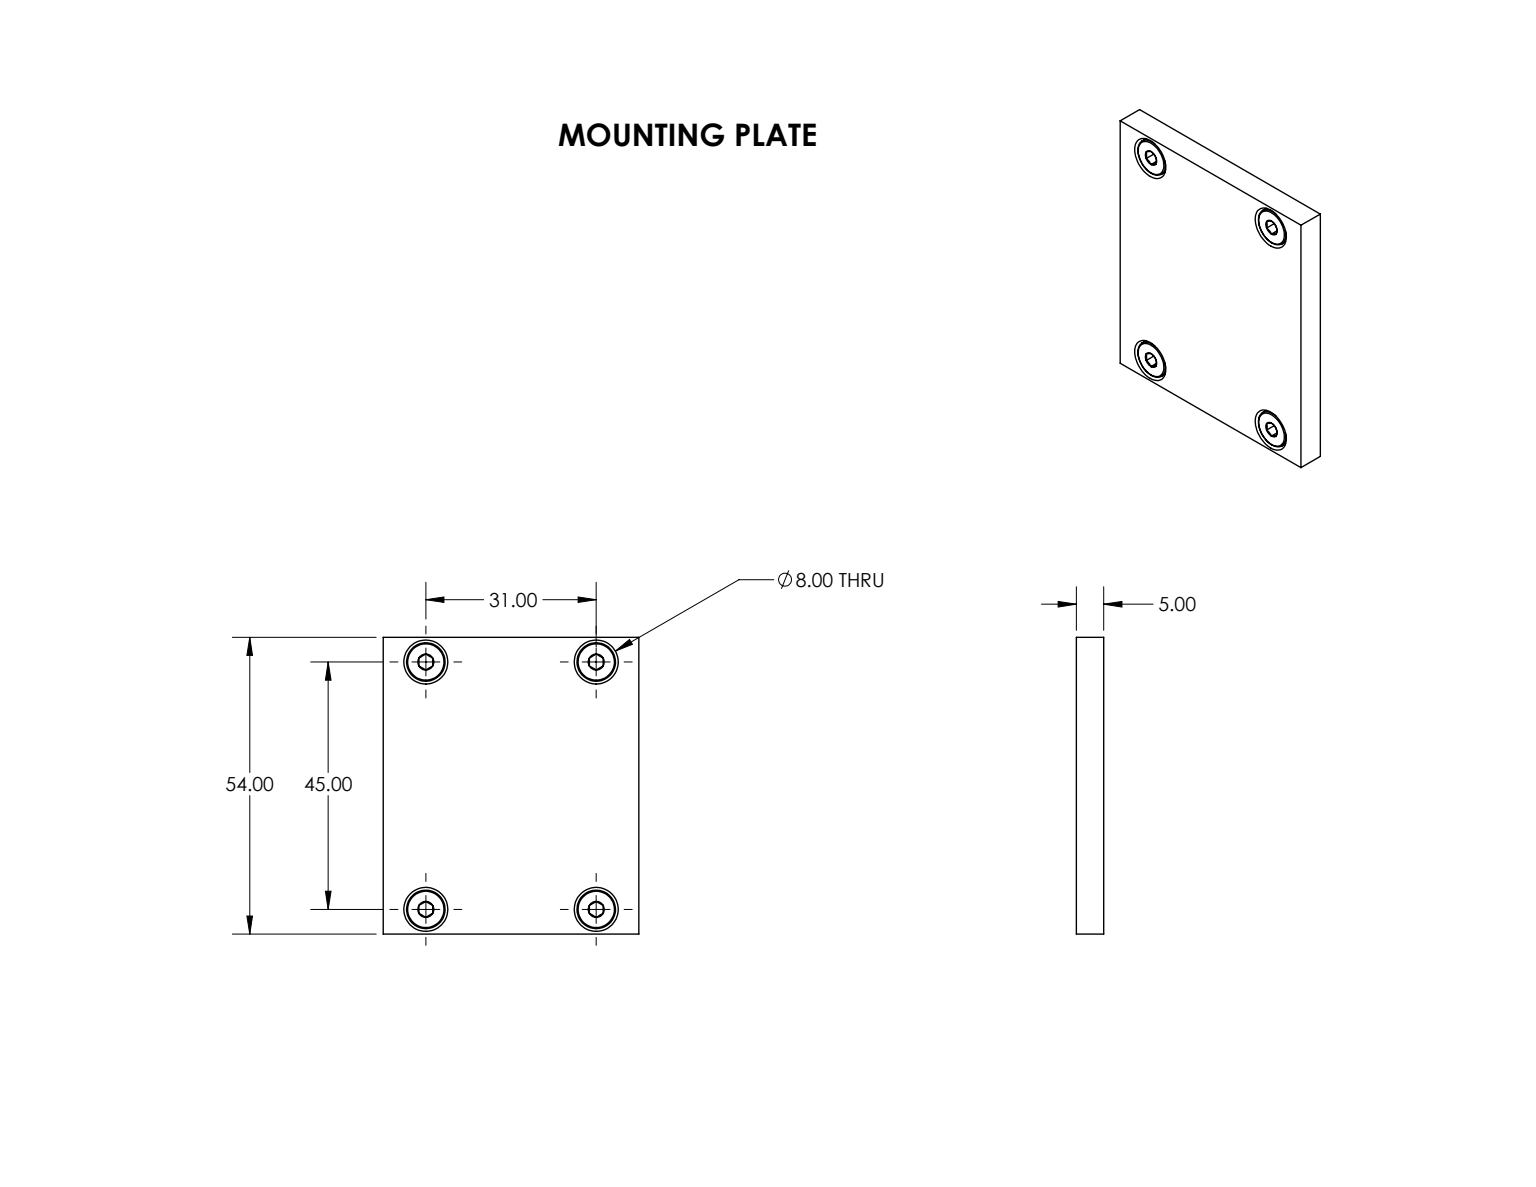
ISO-10303-21;
HEADER;
FILE_DESCRIPTION (('STEP AP214'),
    '1' );
FILE_NAME ('Mounting Plate.step',
    '2026-10-09T17:48:21',
    ( '' ),
    ( '' ),
    'SwSTEP 2.0',
    'SolidWorks 2024',
    '' );
FILE_SCHEMA (( 'AUTOMOTIVE_DESIGN' ));
ENDSEC;

DATA;
#5=CARTESIAN_POINT ( 'NONE',  ( -15.70313394609757296, -0.2715358723600092006, -23.82609623451302028 ) ) ;
#6=DIRECTION ( 'NONE',  ( 0.000000000000000000, 1.000000000000000000, 0.000000000000000000 ) ) ;
#12=DIRECTION ( 'NONE',  ( 0.000000000000000000, 0.000000000000000000, 1.000000000000000000 ) ) ;
#26=CARTESIAN_POINT ( 'NONE',  ( 14.25000000000000000, -0.2038245569916330158, 23.22168783648699986 ) ) ;
#31=CIRCLE ( 'NONE', #14646, 3.499999999999999556 ) ;
#37=ORIENTED_EDGE ( 'NONE', *, *, #9789, .F. ) ;
#41=CARTESIAN_POINT ( 'NONE',  ( 15.50000000000000000, -0.4000000000000000222, -22.50000000000000000 ) ) ;
#49=VECTOR ( 'NONE', #15077, 1000.000000000000000 ) ;
#51=VERTEX_POINT ( 'NONE', #8286 ) ;
#59=VERTEX_POINT ( 'NONE', #14253 ) ;
#64=CARTESIAN_POINT ( 'NONE',  ( -14.25000000000000000, -2.500000000000000000, -23.22168783648699986 ) ) ;
#66=DIRECTION ( 'NONE',  ( -0.8660254037844482555, 0.000000000000000000, 0.4999999999999831801 ) ) ;
#71=VERTEX_POINT ( 'NONE', #12157 ) ;
#76=CARTESIAN_POINT ( 'NONE',  ( -15.91242688423474050, -0.3152598339554945062, -23.70526090034005051 ) ) ;
#77=CARTESIAN_POINT ( 'NONE',  ( 15.50000000000000000, -2.500000000000000000, -21.05662432702600029 ) ) ;
#80=AXIS2_PLACEMENT_3D ( 'NONE', #7760, #5130, #12410 ) ;
#85=CARTESIAN_POINT ( 'NONE',  ( -14.66434062215826017, -0.3156604612126701626, -21.53909249377373669 ) ) ;
#93=AXIS2_PLACEMENT_3D ( 'NONE', #13950, #3324, #14805 ) ;
#96=ORIENTED_EDGE ( 'NONE', *, *, #11121, .T. ) ;
#98=DIRECTION ( 'NONE',  ( 0.000000000000000000, 1.000000000000000000, 0.000000000000000000 ) ) ;
#109=LINE ( 'NONE', #5963, #14166 ) ;
#122=FACE_OUTER_BOUND ( 'NONE', #15028, .T. ) ;
#123=DIRECTION ( 'NONE',  ( 0.000000000000000000, 1.000000000000000000, 0.000000000000000000 ) ) ;
#130=ORIENTED_EDGE ( 'NONE', *, *, #9024, .T. ) ;
#139=CARTESIAN_POINT ( 'NONE',  ( -16.75000000000000000, -2.500000000000000000, -23.22168783648699986 ) ) ;
#146=( NAMED_UNIT ( * ) SI_UNIT ( $, .STERADIAN. ) SOLID_ANGLE_UNIT ( ) );
#150=FACE_OUTER_BOUND ( 'NONE', #9608, .T. ) ;
#154=VECTOR ( 'NONE', #6765, 1000.000000000000000 ) ;
#164=DIRECTION ( 'NONE',  ( -0.9375000000000006661, 0.000000000000000000, -0.3479852726768744020 ) ) ;
#178=DIRECTION ( 'NONE',  ( 0.000000000000000000, 1.000000000000000000, 0.000000000000000000 ) ) ;
#181=VERTEX_POINT ( 'NONE', #14626 ) ;
#183=CARTESIAN_POINT ( 'NONE',  ( -15.50000000000000000, -5.000000000000000000, -22.50000000000000000 ) ) ;
#186=CIRCLE ( 'NONE', #13087, 4.000000000000000000 ) ;
#189=CARTESIAN_POINT ( 'NONE',  ( 15.50000000000000000, -0.4000000000000000222, 25.99999999999999645 ) ) ;
#203=DIRECTION ( 'NONE',  ( 0.000000000000000000, 1.000000000000000000, 0.000000000000000000 ) ) ;
#214=EDGE_CURVE ( 'NONE', #71, #6831, #12240, .T. ) ;
#215=VERTEX_POINT ( 'NONE', #12398 ) ;
#216=CIRCLE ( 'NONE', #8155, 3.499999999999999556 ) ;
#219=CARTESIAN_POINT ( 'NONE',  ( -23.24999999999999645, -5.000000000000000000, 2.987579319737834353E-15 ) ) ;
#240=LINE ( 'NONE', #14588, #11040 ) ;
#252=DIRECTION ( 'NONE',  ( 0.000000000000000000, 1.000000000000000000, 0.000000000000000000 ) ) ;
#253=CYLINDRICAL_SURFACE ( 'NONE', #1029, 4.000000000000000000 ) ;
#254=B_SPLINE_CURVE_WITH_KNOTS ( 'NONE', 3,
 ( #13370, #13070, #7240, #85, #9698, #9626 ),
 .UNSPECIFIED., .F., .F.,
 ( 4, 2, 4 ),
 ( 0.0002380763768129734448, 0.7291065797294584705, 1.457975083082104106 ),
 .UNSPECIFIED. ) ;
#256=DIRECTION ( 'NONE',  ( 0.000000000000000000, 0.000000000000000000, 1.000000000000000000 ) ) ;
#258=ORIENTED_EDGE ( 'NONE', *, *, #13416, .T. ) ;
#266=DIRECTION ( 'NONE',  ( 0.000000000000000000, 1.000000000000000000, 0.000000000000000000 ) ) ;
#272=CARTESIAN_POINT ( 'NONE',  ( 15.50000000000000000, 0.000000000000000000, 22.50000000000000000 ) ) ;
#273=PLANE ( 'NONE',  #3768 ) ;
#278=ORIENTED_EDGE ( 'NONE', *, *, #3265, .F. ) ;
#281=ORIENTED_EDGE ( 'NONE', *, *, #748, .F. ) ;
#285=AXIS2_PLACEMENT_3D ( 'NONE', #3423, #3496, #1409 ) ;
#298=MANIFOLD_SOLID_BREP ( 'Cut-Extrude1[3]', #2333 ) ;
#314=CARTESIAN_POINT ( 'NONE',  ( -15.50000000000000000, -0.4000000000000000222, -22.50000000000000000 ) ) ;
#330=MANIFOLD_SOLID_BREP ( 'Cut-Extrude1[2]', #3578 ) ;
#335=AXIS2_PLACEMENT_3D ( 'NONE', #8151, #10623, #9451 ) ;
#339=EDGE_CURVE ( 'NONE', #3097, #10442, #10612, .T. ) ;
#341=ORIENTED_EDGE ( 'NONE', *, *, #3984, .F. ) ;
#345=EDGE_CURVE ( 'NONE', #11913, #11111, #14089, .T. ) ;
#356=PLANE ( 'NONE',  #3581 ) ;
#363=ORIENTED_EDGE ( 'NONE', *, *, #4204, .F. ) ;
#382=VERTEX_POINT ( 'NONE', #12076 ) ;
#395=( NAMED_UNIT ( * ) SI_UNIT ( $, .STERADIAN. ) SOLID_ANGLE_UNIT ( ) );
#408=VECTOR ( 'NONE', #14676, 1000.000000000000000 ) ;
#412=ORIENTED_EDGE ( 'NONE', *, *, #7830, .T. ) ;
#429=AXIS2_PLACEMENT_3D ( 'NONE', #8275, #13100, #14013 ) ;
#446=DIRECTION ( 'NONE',  ( 0.000000000000000000, 0.000000000000000000, 1.000000000000000000 ) ) ;
#473=DIRECTION ( 'NONE',  ( 0.000000000000000000, 1.000000000000000000, 0.000000000000000000 ) ) ;
#475=PRESENTATION_STYLE_ASSIGNMENT (( #11957 ) ) ;
#481=CARTESIAN_POINT ( 'NONE',  ( -14.25000000000000000, -0.2038245569916330158, 23.22168783648699986 ) ) ;
#490=EDGE_CURVE ( 'NONE', #215, #4608, #7344, .T. ) ;
#496=DIRECTION ( 'NONE',  ( 0.000000000000000000, 1.000000000000000000, 0.000000000000000000 ) ) ;
#500=CARTESIAN_POINT ( 'NONE',  ( 14.25000000000000000, -2.500000000000000000, 23.22168783648699986 ) ) ;
#512=PLANE ( 'NONE',  #4120 ) ;
#523=ORIENTED_EDGE ( 'NONE', *, *, #11573, .T. ) ;
#528=CARTESIAN_POINT ( 'NONE',  ( -15.50000000000000000, -1.037157890325000054, 26.50000000000000000 ) ) ;
#531=FACE_OUTER_BOUND ( 'NONE', #5335, .T. ) ;
#535=DIRECTION ( 'NONE',  ( 0.000000000000000000, 0.000000000000000000, 1.000000000000000000 ) ) ;
#541=VERTEX_POINT ( 'NONE', #8623 ) ;
#544=FACE_OUTER_BOUND ( 'NONE', #4192, .T. ) ;
#552=CARTESIAN_POINT ( 'NONE',  ( -14.25000000000000000, -2.500000000000000000, 23.22168783648699986 ) ) ;
#553=CARTESIAN_POINT ( 'NONE',  ( -15.50000000000000000, -1.037157890325000054, -19.00000000000000000 ) ) ;
#562=CARTESIAN_POINT ( 'NONE',  ( 15.50000000000000000, -1.037157890325000054, -26.50000000000000000 ) ) ;
#579=CIRCLE ( 'NONE', #11243, 1.449999999999996403 ) ;
#580=EDGE_CURVE ( 'NONE', #13163, #4486, #254, .T. ) ;
#581=CIRCLE ( 'NONE', #80, 3.499999999999999556 ) ;
#589=DIRECTION ( 'NONE',  ( 0.000000000000000000, 0.5000000000000199840, 0.8660254037844271613 ) ) ;
#593=AXIS2_PLACEMENT_3D ( 'NONE', #5582, #6516, #11379 ) ;
#594=CARTESIAN_POINT ( 'NONE',  ( 15.50000000000000000, -5.000000000000000000, -19.00000000000000000 ) ) ;
#595=EDGE_CURVE ( 'NONE', #13129, #8137, #10804, .T. ) ;
#608=ORIENTED_EDGE ( 'NONE', *, *, #10263, .T. ) ;
#618=CARTESIAN_POINT ( 'NONE',  ( 14.25000000000000000, -0.2038245569916330158, -21.77831216351300014 ) ) ;
#621=ADVANCED_FACE ( 'NONE', ( #4203 ), #625, .F. ) ;
#625=PLANE ( 'NONE',  #12545 ) ;
#626=PRODUCT_DEFINITION_SHAPE ( 'NONE', 'NONE',  #15168 ) ;
#627=CARTESIAN_POINT ( 'NONE',  ( -15.50000000000000000, -0.2038245569916614930, -21.05662432702600029 ) ) ;
#634=VECTOR ( 'NONE', #10290, 1000.000000000000000 ) ;
#647=DIRECTION ( 'NONE',  ( -0.8660254037844485886, 0.000000000000000000, -0.4999999999999827360 ) ) ;
#649=CARTESIAN_POINT ( 'NONE',  ( 15.50000000000000000, -0.2000000000000000111, 25.80000000297970075 ) ) ;
#650=ORIENTED_EDGE ( 'NONE', *, *, #14893, .F. ) ;
#656=AXIS2_PLACEMENT_3D ( 'NONE', #9390, #1174, #6005 ) ;
#659=LINE ( 'NONE', #5414, #2818 ) ;
#660=CIRCLE ( 'NONE', #12071, 3.499999999999999556 ) ;
#662=DIRECTION ( 'NONE',  ( 0.000000000000000000, 0.000000000000000000, 1.000000000000000000 ) ) ;
#671=ORIENTED_EDGE ( 'NONE', *, *, #799, .F. ) ;
#674=CIRCLE ( 'NONE', #1917, 4.000000000000000000 ) ;
#679=CARTESIAN_POINT ( 'NONE',  ( 15.50000000000000000, -2.500000000000000000, -21.05662432702600029 ) ) ;
#680=CARTESIAN_POINT ( 'NONE',  ( 14.25000000000000000, -2.500000000000000000, -21.77831216351300014 ) ) ;
#687=EDGE_LOOP ( 'NONE', ( #7655, #1654 ) ) ;
#703=CARTESIAN_POINT ( 'NONE',  ( -15.91434062215688350, -0.3156604612129211285, -21.29584399676446793 ) ) ;
#728=ORIENTED_EDGE ( 'NONE', *, *, #5464, .T. ) ;
#733=DIRECTION ( 'NONE',  ( 0.000000000000000000, 0.000000000000000000, 1.000000000000000000 ) ) ;
#736=FACE_OUTER_BOUND ( 'NONE', #12730, .T. ) ;
#747=CARTESIAN_POINT ( 'NONE',  ( 15.50000000000000000, -1.037157890325000054, 22.50000000000000000 ) ) ;
#748=EDGE_CURVE ( 'NONE', #59, #4906, #2885, .T. ) ;
#761=DIRECTION ( 'NONE',  ( 0.000000000000000000, 1.000000000000000000, 0.000000000000000000 ) ) ;
#770=CARTESIAN_POINT ( 'NONE',  ( 16.75000000000000000, -0.2714405302574886547, 22.01253933645462624 ) ) ;
#777=VERTEX_POINT ( 'NONE', #6467 ) ;
#796=STYLED_ITEM ( 'NONE', ( #8444 ), #10531 ) ;
#799=EDGE_CURVE ( 'NONE', #1408, #5494, #8855, .T. ) ;
#805=EDGE_CURVE ( 'NONE', #71, #7389, #9667, .T. ) ;
#808=FACE_OUTER_BOUND ( 'NONE', #14949, .T. ) ;
#823=CARTESIAN_POINT ( 'NONE',  ( -16.94999999999999929, -0.2000000000000000111, -22.50000000000000000 ) ) ;
#825=CARTESIAN_POINT ( 'NONE',  ( 16.75000000000000000, -2.500000000000000000, -23.22168783648699986 ) ) ;
#833=VECTOR ( 'NONE', #8086, 1000.000000000000000 ) ;
#860=DIRECTION ( 'NONE',  ( 0.000000000000000000, 0.000000000000000000, -1.000000000000000000 ) ) ;
#868=DIRECTION ( 'NONE',  ( 0.000000000000000000, 0.000000000000000000, -1.000000000000000000 ) ) ;
#873=EDGE_LOOP ( 'NONE', ( #4886, #278 ) ) ;
#891=FACE_OUTER_BOUND ( 'NONE', #14981, .T. ) ;
#907=FACE_OUTER_BOUND ( 'NONE', #7178, .T. ) ;
#908=DIRECTION ( 'NONE',  ( 0.000000000000000000, 1.000000000000000000, 0.000000000000000000 ) ) ;
#915=ORIENTED_EDGE ( 'NONE', *, *, #5346, .F. ) ;
#931=ORIENTED_EDGE ( 'NONE', *, *, #748, .T. ) ;
#932=CARTESIAN_POINT ( 'NONE',  ( -14.25000000000000000, -0.2038245569916330158, -23.22168783648699986 ) ) ;
#933=ORIENTED_EDGE ( 'NONE', *, *, #4607, .F. ) ;
#938=LINE ( 'NONE', #14971, #4017 ) ;
#960=CARTESIAN_POINT ( 'NONE',  ( 15.50000000000000000, -0.4000000000005274892, -25.79999999999946780 ) ) ;
#961=CARTESIAN_POINT ( 'NONE',  ( -15.50000000000000000, -5.000000000000000000, -26.00000000000000000 ) ) ;
#965=ORIENTED_EDGE ( 'NONE', *, *, #6895, .T. ) ;
#966=DIRECTION ( 'NONE',  ( 0.000000000000000000, -1.000000000000000000, -0.000000000000000000 ) ) ;
#967=EDGE_CURVE ( 'NONE', #10723, #12753, #13779, .T. ) ;
#973=ORIENTED_EDGE ( 'NONE', *, *, #13857, .F. ) ;
#984=PLANE ( 'NONE',  #7031 ) ;
#986=ORIENTED_EDGE ( 'NONE', *, *, #6710, .F. ) ;
#996=FACE_OUTER_BOUND ( 'NONE', #7197, .T. ) ;
#997=EDGE_CURVE ( 'NONE', #8110, #14910, #1607, .T. ) ;
#1009=EDGE_LOOP ( 'NONE', ( #14869, #9513, #7261, #3118 ) ) ;
#1029=AXIS2_PLACEMENT_3D ( 'NONE', #10896, #5000, #9714 ) ;
#1038=CIRCLE ( 'NONE', #9708, 4.000000000000000000 ) ;
#1059=DIRECTION ( 'NONE',  ( 0.000000000000000000, 0.000000000000000000, 1.000000000000000000 ) ) ;
#1070=EDGE_CURVE ( 'NONE', #4318, #8552, #8080, .T. ) ;
#1072=DIRECTION ( 'NONE',  ( 0.000000000000000000, -0.000000000000000000, 1.000000000000000000 ) ) ;
#1073=DIRECTION ( 'NONE',  ( -0.4999999999999832356, 0.000000000000000000, -0.8660254037844483666 ) ) ;
#1075=B_SPLINE_CURVE_WITH_KNOTS ( 'NONE', 3,
 ( #9010, #12658, #3045, #2027, #15050, #12813 ),
 .UNSPECIFIED., .F., .F.,
 ( 4, 2, 4 ),
 ( 0.0002380763768129734448, 0.7291065797294589146, 1.457975083082104995 ),
 .UNSPECIFIED. ) ;
#1094=AXIS2_PLACEMENT_3D ( 'NONE', #12697, #4639, #6961 ) ;
#1095=EDGE_CURVE ( 'NONE', #11388, #11166, #13173, .T. ) ;
#1099=CARTESIAN_POINT ( 'NONE',  ( -14.25000000000000000, -0.2038245569916330158, 23.22168783648699986 ) ) ;
#1102=CARTESIAN_POINT ( 'NONE',  ( 16.75000000000000000, -2.500000000000000000, 21.77831216351300014 ) ) ;
#1109=ORIENTED_EDGE ( 'NONE', *, *, #4097, .F. ) ;
#1112=EDGE_CURVE ( 'NONE', #4275, #181, #10269, .T. ) ;
#1114=VERTEX_POINT ( 'NONE', #12546 ) ;
#1116=CARTESIAN_POINT ( 'NONE',  ( 15.50000000000000000, 0.000000000000000000, -22.50000000000000000 ) ) ;
#1118=AXIS2_PLACEMENT_3D ( 'NONE', #3027, #10142, #13735 ) ;
#1120=VECTOR ( 'NONE', #11401, 1000.000000000000000 ) ;
#1141=DIRECTION ( 'NONE',  ( 0.000000000000000000, 1.000000000000000000, 0.000000000000000000 ) ) ;
#1146=ORIENTED_EDGE ( 'NONE', *, *, #9815, .F. ) ;
#1150=EDGE_LOOP ( 'NONE', ( #965, #3065, #8473, #1387, #1741, #5883 ) ) ;
#1152=VECTOR ( 'NONE', #13066, 1000.000000000000000 ) ;
#1161=EDGE_CURVE ( 'NONE', #6610, #6972, #7948, .T. ) ;
#1166=CARTESIAN_POINT ( 'NONE',  ( -14.45313394609757118, -0.2715358723599894386, -23.33896727494798284 ) ) ;
#1168=ORIENTED_EDGE ( 'NONE', *, *, #4774, .F. ) ;
#1169=ORIENTED_EDGE ( 'NONE', *, *, #7747, .F. ) ;
#1173=EDGE_CURVE ( 'NONE', #1706, #5891, #11563, .T. ) ;
#1174=DIRECTION ( 'NONE',  ( -1.000000000000000000, 0.000000000000000000, 0.000000000000000000 ) ) ;
#1184=VERTEX_POINT ( 'NONE', #12393 ) ;
#1211=LINE ( 'NONE', #5970, #14749 ) ;
#1217=PLANE ( 'NONE',  #12937 ) ;
#1228=CARTESIAN_POINT ( 'NONE',  ( -30.00000000000000000, -5.000000000000000000, 27.00000000000000000 ) ) ;
#1229=DIRECTION ( 'NONE',  ( -0.000000000000000000, 1.000000000000000000, 0.000000000000000000 ) ) ;
#1246=LINE ( 'NONE', #4832, #3529 ) ;
#1254=ORIENTED_EDGE ( 'NONE', *, *, #1173, .F. ) ;
#1264=CARTESIAN_POINT ( 'NONE',  ( -16.33565937784310762, -0.3156604612129118026, 21.53909249377453250 ) ) ;
#1267=AXIS2_PLACEMENT_3D ( 'NONE', #823, #11377, #6737 ) ;
#1279=ORIENTED_EDGE ( 'NONE', *, *, #2419, .F. ) ;
#1280=AXIS2_PLACEMENT_3D ( 'NONE', #10048, #1980, #4088 ) ;
#1289=CARTESIAN_POINT ( 'NONE',  ( 14.25000000000000000, -2.500000000000000000, 23.22168783648699986 ) ) ;
#1309=FILL_AREA_STYLE ('',( #6070 ) ) ;
#1316=EDGE_LOOP ( 'NONE', ( #6456, #4036, #931, #1168 ) ) ;
#1318=ORIENTED_EDGE ( 'NONE', *, *, #12388, .T. ) ;
#1322=CARTESIAN_POINT ( 'NONE',  ( 15.50000000000000000, -5.000000000000000000, 22.50000000000000000 ) ) ;
#1324=AXIS2_PLACEMENT_3D ( 'NONE', #14681, #1434, #256 ) ;
#1332=CARTESIAN_POINT ( 'NONE',  ( -14.25000000000000000, -2.500000000000000000, 23.22168783648699986 ) ) ;
#1335=EDGE_CURVE ( 'NONE', #14415, #13870, #660, .T. ) ;
#1340=CLOSED_SHELL ( 'NONE', ( #1484, #14239, #7741, #10570, #14326, #4894, #5553, #4994, #9912, #11153, #4510, #6147, #11998, #6486 ) ) ;
#1359=EDGE_CURVE ( 'NONE', #3822, #12945, #13090, .T. ) ;
#1362=VECTOR ( 'NONE', #3810, 1000.000000000000000 ) ;
#1368=CARTESIAN_POINT ( 'NONE',  ( 14.25000000000000000, -2.500000000000000000, 21.77831216351300014 ) ) ;
#1387=ORIENTED_EDGE ( 'NONE', *, *, #1161, .T. ) ;
#1392=VECTOR ( 'NONE', #2531, 1000.000000000000000 ) ;
#1394=CARTESIAN_POINT ( 'NONE',  ( -15.50000000000000000, -5.000000000000000000, 19.00000000000000000 ) ) ;
#1408=VERTEX_POINT ( 'NONE', #5169 ) ;
#1409=DIRECTION ( 'NONE',  ( 1.000000000000000000, 0.000000000000000000, 0.000000000000000000 ) ) ;
#1418=FACE_OUTER_BOUND ( 'NONE', #5044, .T. ) ;
#1423=ORIENTED_EDGE ( 'NONE', *, *, #1112, .F. ) ;
#1424=ORIENTED_EDGE ( 'NONE', *, *, #4905, .F. ) ;
#1425=CARTESIAN_POINT ( 'NONE',  ( 15.50000000000000000, -0.2000000000000000111, 19.19999999702029925 ) ) ;
#1434=DIRECTION ( 'NONE',  ( 0.000000000000000000, -1.000000000000000000, -0.000000000000000000 ) ) ;
#1438=ORIENTED_EDGE ( 'NONE', *, *, #8297, .F. ) ;
#1439=DIRECTION ( 'NONE',  ( 0.000000000000000000, 1.000000000000000000, 0.000000000000000000 ) ) ;
#1443=EDGE_LOOP ( 'NONE', ( #933, #5709, #3137, #8529 ) ) ;
#1467=CIRCLE ( 'NONE', #10121, 3.499999999999999556 ) ;
#1476=ORIENTED_EDGE ( 'NONE', *, *, #3651, .F. ) ;
#1479=ADVANCED_FACE ( 'NONE', ( #2743 ), #8837, .T. ) ;
#1484=ADVANCED_FACE ( 'NONE', ( #8417 ), #13159, .F. ) ;
#1485=DIRECTION ( 'NONE',  ( 0.000000000000000000, 1.000000000000000000, 0.000000000000000000 ) ) ;
#1495=DIRECTION ( 'NONE',  ( 0.3479852726768751237, 0.000000000000000000, -0.9375000000000004441 ) ) ;
#1511=ORIENTED_EDGE ( 'NONE', *, *, #2723, .F. ) ;
#1512=VECTOR ( 'NONE', #13696, 1000.000000000000000 ) ;
#1519=CARTESIAN_POINT ( 'NONE',  ( -15.50000000000000000, -0.4000000000000000222, -19.00000000000000355 ) ) ;
#1522=PLANE ( 'NONE',  #10361 ) ;
#1528=VERTEX_POINT ( 'NONE', #189 ) ;
#1539=DIRECTION ( 'NONE',  ( 0.000000000000000000, 1.000000000000000000, 0.000000000000000000 ) ) ;
#1540=AXIS2_PLACEMENT_3D ( 'NONE', #14942, #4334, #13798 ) ;
#1551=VERTEX_POINT ( 'NONE', #649 ) ;
#1553=EDGE_CURVE ( 'NONE', #15023, #5866, #5990, .T. ) ;
#1559=CARTESIAN_POINT ( 'NONE',  ( 16.33757311576526305, -0.3152598339554795182, 21.54019739087904384 ) ) ;
#1607=LINE ( 'NONE', #5184, #9066 ) ;
#1610=EDGE_LOOP ( 'NONE', ( #8334, #14233 ) ) ;
#1620=PLANE ( 'NONE',  #12693 ) ;
#1628=VERTEX_POINT ( 'NONE', #500 ) ;
#1633=TOROIDAL_SURFACE ( 'NONE', #7823, 3.299999999999474909, 0.2000000000005234813 ) ;
#1635=AXIS2_PLACEMENT_3D ( 'NONE', #11045, #4929, #12135 ) ;
#1647=CARTESIAN_POINT ( 'NONE',  ( 16.75000000000000000, -0.2038245569916320166, -21.77831216351300014 ) ) ;
#1654=ORIENTED_EDGE ( 'NONE', *, *, #9802, .T. ) ;
#1663=LINE ( 'NONE', #562, #8572 ) ;
#1669=ORIENTED_EDGE ( 'NONE', *, *, #15306, .T. ) ;
#1678=CARTESIAN_POINT ( 'NONE',  ( 15.50000000000000000, -1.037157890325000054, -18.50000000000000000 ) ) ;
#1681=AXIS2_PLACEMENT_3D ( 'NONE', #2035, #8163, #9320 ) ;
#1684=CARTESIAN_POINT ( 'NONE',  ( 16.75000000000000000, -0.2038245569916320166, 23.22168783648699986 ) ) ;
#1694=CARTESIAN_POINT ( 'NONE',  ( -16.75000000000000000, -2.500000000000000000, 23.22168783648699986 ) ) ;
#1695=LINE ( 'NONE', #528, #14945 ) ;
#1697=LINE ( 'NONE', #14570, #8886 ) ;
#1698=DIRECTION ( 'NONE',  ( 0.9375000000000004441, 0.000000000000000000, 0.3479852726768752902 ) ) ;
#1699=CARTESIAN_POINT ( 'NONE',  ( 16.75000000000000000, -2.500000000000000000, -23.22168783648699986 ) ) ;
#1706=VERTEX_POINT ( 'NONE', #14214 ) ;
#1712=CARTESIAN_POINT ( 'NONE',  ( 14.25000000000000178, -0.2714405302574905421, -22.01253933645463690 ) ) ;
#1713=CARTESIAN_POINT ( 'NONE',  ( 15.70366306705349757, -0.2717122460102775472, 21.17420925361331641 ) ) ;
#1715=CARTESIAN_POINT ( 'NONE',  ( -15.50000000000000000, -5.000000000000000000, 18.50000000000000000 ) ) ;
#1717=DIRECTION ( 'NONE',  ( 0.000000000000000000, 0.000000000000000000, 1.000000000000000000 ) ) ;
#1741=ORIENTED_EDGE ( 'NONE', *, *, #10652, .T. ) ;
#1771=CARTESIAN_POINT ( 'NONE',  ( -15.50000000000000000, -0.2038245569916614930, 23.94337567297399971 ) ) ;
#1779=CARTESIAN_POINT ( 'NONE',  ( -15.50000000000000000, -1.037157890325000054, 26.00000000000000000 ) ) ;
#1782=DIRECTION ( 'NONE',  ( 0.000000000000000000, 0.000000000000000000, 1.000000000000000000 ) ) ;
#1796=ORIENTED_EDGE ( 'NONE', *, *, #490, .F. ) ;
#1810=EDGE_CURVE ( 'NONE', #2099, #14169, #6864, .T. ) ;
#1812=CIRCLE ( 'NONE', #8000, 4.000000000000000000 ) ;
#1825=DIRECTION ( 'NONE',  ( 0.000000000000000000, -1.000000000000000000, -0.000000000000000000 ) ) ;
#1829=LINE ( 'NONE', #4240, #2275 ) ;
#1843=CYLINDRICAL_SURFACE ( 'NONE', #13932, 4.000000000000000000 ) ;
#1844=CARTESIAN_POINT ( 'NONE',  ( -14.25000000000000000, -0.2038245569916330158, -21.77831216351300014 ) ) ;
#1850=EDGE_LOOP ( 'NONE', ( #8013, #13009, #13275, #13946 ) ) ;
#1852=ORIENTED_EDGE ( 'NONE', *, *, #5042, .F. ) ;
#1853=ORIENTED_EDGE ( 'NONE', *, *, #1810, .F. ) ;
#1855=VERTEX_POINT ( 'NONE', #8626 ) ;
#1871=CARTESIAN_POINT ( 'NONE',  ( 16.75000000000000355, -0.2715193793361441177, 22.98718409945082897 ) ) ;
#1873=CARTESIAN_POINT ( 'NONE',  ( -15.50000000000000000, -2.500000000000000000, -23.94337567297399971 ) ) ;
#1885=B_SPLINE_CURVE_WITH_KNOTS ( 'NONE', 3,
 ( #12579, #10078, #12349, #14658, #1712, #618 ),
 .UNSPECIFIED., .F., .F.,
 ( 4, 2, 4 ),
 ( 1.820537833122031657, 2.555393473688635897, 3.290249114255240137 ),
 .UNSPECIFIED. ) ;
#1904=CARTESIAN_POINT ( 'NONE',  ( 14.25000000000000000, -0.3156864504677177052, 22.25638000318208753 ) ) ;
#1915=VERTEX_POINT ( 'NONE', #13216 ) ;
#1916=EDGE_CURVE ( 'NONE', #6810, #5926, #9087, .T. ) ;
#1917=AXIS2_PLACEMENT_3D ( 'NONE', #7126, #12857, #11684 ) ;
#1937=EDGE_CURVE ( 'NONE', #12753, #10723, #4388, .T. ) ;
#1961=VECTOR ( 'NONE', #5648, 1000.000000000000000 ) ;
#1969=CARTESIAN_POINT ( 'NONE',  ( -15.50000000000000000, -0.4000000000000000222, 25.99999999999999645 ) ) ;
#1974=FACE_OUTER_BOUND ( 'NONE', #5634, .T. ) ;
#1979=DIRECTION ( 'NONE',  ( 0.000000000000000000, -1.000000000000000000, -0.000000000000000000 ) ) ;
#1980=DIRECTION ( 'NONE',  ( 1.000000000000000000, 0.000000000000000000, 0.000000000000000000 ) ) ;
#1999=ORIENTED_EDGE ( 'NONE', *, *, #580, .T. ) ;
#2001=EDGE_LOOP ( 'NONE', ( #728, #12873 ) ) ;
#2017=ORIENTED_EDGE ( 'NONE', *, *, #2580, .F. ) ;
#2025=UNCERTAINTY_MEASURE_WITH_UNIT (LENGTH_MEASURE( 1.000000000000000082E-05 ), #8770, 'distance_accuracy_value', 'NONE');
#2027=CARTESIAN_POINT ( 'NONE',  ( 16.33565937784172917, -0.3156604612126656106, 23.46090750622625976 ) ) ;
#2035=CARTESIAN_POINT ( 'NONE',  ( -15.50000000000000000, -5.000000000000000000, 22.50000000000000000 ) ) ;
#2052=EDGE_CURVE ( 'NONE', #9286, #14331, #10155, .T. ) ;
#2053=CARTESIAN_POINT ( 'NONE',  ( 15.50000000000000000, -1.037157890325000054, 22.50000000000000000 ) ) ;
#2054=CARTESIAN_POINT ( 'NONE',  ( 15.50000000000000000, -0.4000000000005274892, -22.50000000000000000 ) ) ;
#2060=FACE_OUTER_BOUND ( 'NONE', #6283, .T. ) ;
#2072=DIRECTION ( 'NONE',  ( 0.000000000000000000, 0.000000000000000000, 1.000000000000000000 ) ) ;
#2076=VECTOR ( 'NONE', #5809, 1000.000000000000000 ) ;
#2082=EDGE_LOOP ( 'NONE', ( #9067, #9804, #5693, #973 ) ) ;
#2092=DIRECTION ( 'NONE',  ( 0.000000000000000000, 0.000000000000000000, 1.000000000000000000 ) ) ;
#2099=VERTEX_POINT ( 'NONE', #1873 ) ;
#2110=LINE ( 'NONE', #5855, #13817 ) ;
#2112=MECHANICAL_DESIGN_GEOMETRIC_PRESENTATION_REPRESENTATION('',(#8805),#4597);
#2116=AXIS2_PLACEMENT_3D ( 'NONE', #14941, #2942, #6600 ) ;
#2121=EDGE_LOOP ( 'NONE', ( #11341, #8950, #258, #8862 ) ) ;
#2130=FACE_OUTER_BOUND ( 'NONE', #9678, .T. ) ;
#2134=AXIS2_PLACEMENT_3D ( 'NONE', #272, #5109, #13480 ) ;
#2136=CARTESIAN_POINT ( 'NONE',  ( -15.50000000000000000, 998.9628421096749662, 22.50000000000000000 ) ) ;
#2143=EDGE_CURVE ( 'NONE', #8110, #10442, #14120, .T. ) ;
#2153=ORIENTED_EDGE ( 'NONE', *, *, #14095, .T. ) ;
#2156=AXIS2_PLACEMENT_3D ( 'NONE', #15240, #2293, #4552 ) ;
#2160=ORIENTED_EDGE ( 'NONE', *, *, #7553, .T. ) ;
#2164=CARTESIAN_POINT ( 'NONE',  ( 14.25000000000000000, -2.500000000000000000, 21.77831216351300014 ) ) ;
#2168=LINE ( 'NONE', #7071, #2279 ) ;
#2177=EDGE_CURVE ( 'NONE', #13870, #11017, #9224, .T. ) ;
#2182=CARTESIAN_POINT ( 'NONE',  ( -16.54633693294649888, -0.2717122460102565085, -23.33927276307431598 ) ) ;
#2190=AXIS2_PLACEMENT_3D ( 'NONE', #4181, #2941, #12103 ) ;
#2193=EDGE_CURVE ( 'NONE', #2946, #9156, #3355, .T. ) ;
#2237=LINE ( 'NONE', #7911, #4287 ) ;
#2239=CARTESIAN_POINT ( 'NONE',  ( -15.50000000000000000, -0.4000000000000000222, -25.99999999999999645 ) ) ;
#2240=DIRECTION ( 'NONE',  ( 0.000000000000000000, 1.000000000000000000, 0.000000000000000000 ) ) ;
#2241=CARTESIAN_POINT ( 'NONE',  ( -16.75000000000000000, -0.2038245569916330158, 21.77831216351300014 ) ) ;
#2252=( NAMED_UNIT ( * ) SI_UNIT ( $, .STERADIAN. ) SOLID_ANGLE_UNIT ( ) );
#2257=DIRECTION ( 'NONE',  ( -1.284980352575412699E-16, 0.000000000000000000, -1.000000000000000000 ) ) ;
#2259=PLANE ( 'NONE',  #7881 ) ;
#2268=CARTESIAN_POINT ( 'NONE',  ( -16.75000000000000000, -0.2038245569916330158, -23.22168783648699986 ) ) ;
#2269=ORIENTED_EDGE ( 'NONE', *, *, #4403, .T. ) ;
#2275=VECTOR ( 'NONE', #6662, 1000.000000000000000 ) ;
#2279=VECTOR ( 'NONE', #2240, 1000.000000000000000 ) ;
#2287=PRESENTATION_STYLE_ASSIGNMENT (( #4466 ) ) ;
#2293=DIRECTION ( 'NONE',  ( 0.000000000000000000, 1.000000000000000000, 0.000000000000000000 ) ) ;
#2298=DIRECTION ( 'NONE',  ( 0.000000000000000000, 0.000000000000000000, 1.000000000000000000 ) ) ;
#2302=CARTESIAN_POINT ( 'NONE',  ( 23.25000000000000000, -10.00000000000000000, 27.00000000000000000 ) ) ;
#2308=EDGE_LOOP ( 'NONE', ( #8118, #3549, #10138, #7854 ) ) ;
#2311=ORIENTED_EDGE ( 'NONE', *, *, #3453, .F. ) ;
#2333=CLOSED_SHELL ( 'NONE', ( #11664, #4399, #12367, #12302, #7256, #5871, #621, #2702, #12849, #14914, #5915, #7560, #7065, #8954, #10860 ) ) ;
#2334=VECTOR ( 'NONE', #473, 1000.000000000000000 ) ;
#2338=CARTESIAN_POINT ( 'NONE',  ( 15.29686605390242704, -0.2715358723600077573, 21.17390376548697972 ) ) ;
#2341=DIRECTION ( 'NONE',  ( 0.000000000000000000, 1.000000000000000000, 0.000000000000000000 ) ) ;
#2344=FACE_BOUND ( 'NONE', #12322, .T. ) ;
#2356=FACE_OUTER_BOUND ( 'NONE', #8011, .T. ) ;
#2380=FACE_OUTER_BOUND ( 'NONE', #7641, .T. ) ;
#2384=ORIENTED_EDGE ( 'NONE', *, *, #9675, .F. ) ;
#2389=AXIS2_PLACEMENT_3D ( 'NONE', #12300, #2593, #3760 ) ;
#2416=LINE ( 'NONE', #9391, #12683 ) ;
#2419=EDGE_CURVE ( 'NONE', #10261, #13163, #6227, .T. ) ;
#2422=DIRECTION ( 'NONE',  ( 0.000000000000000000, 1.000000000000000000, 0.000000000000000000 ) ) ;
#2440=CARTESIAN_POINT ( 'NONE',  ( -15.50000000000000000, -0.2038245569916614930, -23.94337567297399971 ) ) ;
#2454=CARTESIAN_POINT ( 'NONE',  ( -15.50000000000000000, -0.4000000000005236034, -19.20000000000052509 ) ) ;
#2458=ORIENTED_EDGE ( 'NONE', *, *, #2913, .F. ) ;
#2464=DIRECTION ( 'NONE',  ( 1.000000000000000000, 0.000000000000000000, 0.000000000000000000 ) ) ;
#2468=APPLICATION_CONTEXT ( 'automotive_design' ) ;
#2470=DIRECTION ( 'NONE',  ( -0.4999999999999832356, 0.000000000000000000, 0.8660254037844483666 ) ) ;
#2471=PLANE ( 'NONE',  #9798 ) ;
#2472=ADVANCED_FACE ( 'NONE', ( #3017, #6378 ), #2867, .T. ) ;
#2476=B_SPLINE_CURVE_WITH_KNOTS ( 'NONE', 3,
 ( #14449, #11981, #3604, #1264, #8561, #3681 ),
 .UNSPECIFIED., .F., .F.,
 ( 4, 2, 4 ),
 ( 0.0002380763768129734448, 0.7291065797294591366, 1.457975083082105439 ),
 .UNSPECIFIED. ) ;
#2477=DIRECTION ( 'NONE',  ( 0.000000000000000000, 1.000000000000000000, 0.000000000000000000 ) ) ;
#2487=CYLINDRICAL_SURFACE ( 'NONE', #8585, 3.499999999999999556 ) ;
#2488=DIRECTION ( 'NONE',  ( -0.8660254037844482555, 0.000000000000000000, 0.4999999999999831801 ) ) ;
#2489=DIRECTION ( 'NONE',  ( 0.000000000000000000, 1.000000000000000000, 0.000000000000000000 ) ) ;
#2498=FACE_OUTER_BOUND ( 'NONE', #8881, .T. ) ;
#2505=EDGE_CURVE ( 'NONE', #382, #14751, #581, .T. ) ;
#2515=DIRECTION ( 'NONE',  ( 0.8660254037844482555, 0.000000000000000000, 0.4999999999999831801 ) ) ;
#2519=EDGE_CURVE ( 'NONE', #7520, #3938, #12234, .T. ) ;
#2524=ADVANCED_FACE ( 'NONE', ( #13649 ), #14644, .F. ) ;
#2525=DIRECTION ( 'NONE',  ( 0.000000000000000000, 1.000000000000000000, 0.000000000000000000 ) ) ;
#2531=DIRECTION ( 'NONE',  ( 0.000000000000000000, 1.000000000000000000, 0.000000000000000000 ) ) ;
#2544=VECTOR ( 'NONE', #13814, 999.9999999999998863 ) ;
#2550=DIRECTION ( 'NONE',  ( 0.000000000000000000, 1.000000000000000000, 0.000000000000000000 ) ) ;
#2553=DIRECTION ( 'NONE',  ( 0.000000000000000000, 0.000000000000000000, 1.000000000000000000 ) ) ;
#2572=CYLINDRICAL_SURFACE ( 'NONE', #12702, 3.499999999999999556 ) ;
#2580=EDGE_CURVE ( 'NONE', #6830, #7739, #8711, .T. ) ;
#2593=DIRECTION ( 'NONE',  ( 0.000000000000000000, 1.000000000000000000, 0.000000000000000000 ) ) ;
#2600=EDGE_CURVE ( 'NONE', #541, #11427, #6524, .T. ) ;
#2608=CYLINDRICAL_SURFACE ( 'NONE', #4435, 3.499999999999999556 ) ;
#2610=CARTESIAN_POINT ( 'NONE',  ( 15.50000000000000000, -0.2000000000000000111, -22.50000000000000000 ) ) ;
#2612=CARTESIAN_POINT ( 'NONE',  ( -15.50000000000000000, -0.2000000000000000111, 22.50000000000000000 ) ) ;
#2617=AXIS2_PLACEMENT_3D ( 'NONE', #2863, #7610, #1698 ) ;
#2625=EDGE_CURVE ( 'NONE', #7520, #10300, #10368, .T. ) ;
#2646=CARTESIAN_POINT ( 'NONE',  ( 30.00000000000000000, 0.000000000000000000, -27.00000000000000000 ) ) ;
#2656=DIRECTION ( 'NONE',  ( 0.000000000000000000, 1.000000000000000000, 0.000000000000000000 ) ) ;
#2702=ADVANCED_FACE ( 'NONE', ( #11385 ), #984, .F. ) ;
#2709=CARTESIAN_POINT ( 'NONE',  ( -15.50000000000000000, -0.2000000000000000111, 19.20000000000052509 ) ) ;
#2711=CARTESIAN_POINT ( 'NONE',  ( 15.50000000000000000, -1.037157890325000054, 22.50000000000000000 ) ) ;
#2712=ADVANCED_FACE ( 'NONE', ( #3168 ), #10439, .F. ) ;
#2717=ORIENTED_EDGE ( 'NONE', *, *, #4485, .F. ) ;
#2723=EDGE_CURVE ( 'NONE', #3944, #4925, #8518, .T. ) ;
#2727=DIRECTION ( 'NONE',  ( 0.000000000000000000, 1.000000000000000000, 0.000000000000000000 ) ) ;
#2728=CARTESIAN_POINT ( 'NONE',  ( 16.75000000000000000, -0.2038245569916320166, -23.22168783648699986 ) ) ;
#2729=ORIENTED_EDGE ( 'NONE', *, *, #15169, .T. ) ;
#2740=DIRECTION ( 'NONE',  ( 0.000000000000000000, -1.000000000000000000, -0.000000000000000000 ) ) ;
#2743=FACE_OUTER_BOUND ( 'NONE', #12732, .T. ) ;
#2745=AXIS2_PLACEMENT_3D ( 'NONE', #41, #266, #7585 ) ;
#2779=FACE_OUTER_BOUND ( 'NONE', #5317, .T. ) ;
#2787=ORIENTED_EDGE ( 'NONE', *, *, #8789, .F. ) ;
#2792=ORIENTED_EDGE ( 'NONE', *, *, #11668, .T. ) ;
#2796=AXIS2_PLACEMENT_3D ( 'NONE', #3859, #12153, #7436 ) ;
#2797=( NAMED_UNIT ( * ) PLANE_ANGLE_UNIT ( ) SI_UNIT ( $, .RADIAN. ) );
#2800=CARTESIAN_POINT ( 'NONE',  ( 16.75000000000000000, -0.2038245569916320166, 21.77831216351300014 ) ) ;
#2815=UNCERTAINTY_MEASURE_WITH_UNIT (LENGTH_MEASURE( 1.000000000000000082E-05 ), #7825, 'distance_accuracy_value', 'NONE');
#2817=EDGE_CURVE ( 'NONE', #4608, #5722, #13107, .T. ) ;
#2818=VECTOR ( 'NONE', #8960, 1000.000000000000000 ) ;
#2824=PLANE ( 'NONE',  #12582 ) ;
#2829=AXIS2_PLACEMENT_3D ( 'NONE', #10249, #12600, #7866 ) ;
#2838=AXIS2_PLACEMENT_3D ( 'NONE', #9242, #13980, #10250 ) ;
#2857=PLANE ( 'NONE',  #6877 ) ;
#2862=AXIS2_PLACEMENT_3D ( 'NONE', #2454, #15163, #2298 ) ;
#2863=CARTESIAN_POINT ( 'NONE',  ( -15.50000000000000000, -5.000000000000000000, 22.50000000000000000 ) ) ;
#2865=DIRECTION ( 'NONE',  ( -0.8660254037844482555, 0.000000000000000000, -0.4999999999999831801 ) ) ;
#2867=PLANE ( 'NONE',  #13235 ) ;
#2877=CIRCLE ( 'NONE', #14262, 0.2000000000005261458 ) ;
#2879=PLANE ( 'NONE',  #1118 ) ;
#2881=PLANE ( 'NONE',  #10978 ) ;
#2885=CIRCLE ( 'NONE', #5884, 0.2000000000005261458 ) ;
#2894=ORIENTED_EDGE ( 'NONE', *, *, #12670, .F. ) ;
#2901=VECTOR ( 'NONE', #2959, 1000.000000000000000 ) ;
#2906=LINE ( 'NONE', #10100, #15025 ) ;
#2912=CARTESIAN_POINT ( 'NONE',  ( 15.50000000000000000, -0.2038245569916604938, 23.94337567297399971 ) ) ;
#2913=EDGE_CURVE ( 'NONE', #11111, #14331, #14478, .T. ) ;
#2916=ORIENTED_EDGE ( 'NONE', *, *, #8205, .T. ) ;
#2921=DIRECTION ( 'NONE',  ( -0.8660254037844482555, 0.000000000000000000, 0.4999999999999831801 ) ) ;
#2925=DIRECTION ( 'NONE',  ( -0.000000000000000000, 1.000000000000000000, 0.000000000000000000 ) ) ;
#2926=CARTESIAN_POINT ( 'NONE',  ( 30.00000000000000000, -5.000000000000000000, -27.00000000000000000 ) ) ;
#2929=SHAPE_REPRESENTATION ( 'Mounting Plate', ( #285 ), #14401 ) ;
#2930=EDGE_LOOP ( 'NONE', ( #412, #5424, #10019, #11721 ) ) ;
#2939=CARTESIAN_POINT ( 'NONE',  ( -16.75000000000000000, -0.2038245569916330158, 23.22168783648699986 ) ) ;
#2940=CONICAL_SURFACE ( 'NONE', #2190, 1732.050807568789651, 1.047197551196575871 ) ;
#2941=DIRECTION ( 'NONE',  ( 0.000000000000000000, 1.000000000000000000, 0.000000000000000000 ) ) ;
#2942=DIRECTION ( 'NONE',  ( -0.4999999999999832356, 0.000000000000000000, -0.8660254037844483666 ) ) ;
#2946=VERTEX_POINT ( 'NONE', #7133 ) ;
#2947=ORIENTED_EDGE ( 'NONE', *, *, #5042, .T. ) ;
#2948=ORIENTED_EDGE ( 'NONE', *, *, #11668, .F. ) ;
#2952=CARTESIAN_POINT ( 'NONE',  ( 15.50000000000000000, -2.500000000000000000, -21.05662432702600029 ) ) ;
#2959=DIRECTION ( 'NONE',  ( 0.000000000000000000, 0.000000000000000000, 1.000000000000000000 ) ) ;
#2965=ORIENTED_EDGE ( 'NONE', *, *, #9901, .F. ) ;
#2966=DIRECTION ( 'NONE',  ( -0.000000000000000000, -0.000000000000000000, 1.000000000000000000 ) ) ;
#2970=UNCERTAINTY_MEASURE_WITH_UNIT (LENGTH_MEASURE( 1.000000000000000082E-05 ), #10862, 'distance_accuracy_value', 'NONE');
#2998=CARTESIAN_POINT ( 'NONE',  ( 15.50000000000000000, -0.4000000000005274892, 19.20000000000052864 ) ) ;
#3014=FACE_OUTER_BOUND ( 'NONE', #9328, .T. ) ;
#3017=FACE_OUTER_BOUND ( 'NONE', #5013, .T. ) ;
#3019=CIRCLE ( 'NONE', #4001, 0.2000000000005261458 ) ;
#3023=VERTEX_POINT ( 'NONE', #11007 ) ;
#3027=CARTESIAN_POINT ( 'NONE',  ( 0.000000000000000000, 0.000000000000000000, 0.000000000000000000 ) ) ;
#3037=ORIENTED_EDGE ( 'NONE', *, *, #2052, .F. ) ;
#3042=VERTEX_POINT ( 'NONE', #14337 ) ;
#3045=CARTESIAN_POINT ( 'NONE',  ( 15.91242688423647955, -0.3152598339557988183, 23.70526090033903799 ) ) ;
#3055=VERTEX_POINT ( 'NONE', #1394 ) ;
#3059=DIRECTION ( 'NONE',  ( 0.8660254037844482555, 0.000000000000000000, 0.4999999999999831801 ) ) ;
#3065=ORIENTED_EDGE ( 'NONE', *, *, #12568, .T. ) ;
#3066=CARTESIAN_POINT ( 'NONE',  ( 15.50000000000000000, -0.1999999999999999556, -23.94999999999999574 ) ) ;
#3067=CARTESIAN_POINT ( 'NONE',  ( -15.50000000000000000, -2.500000000000000000, 23.94337567297399971 ) ) ;
#3069=AXIS2_PLACEMENT_3D ( 'NONE', #8636, #2740, #3983 ) ;
#3083=ORIENTED_EDGE ( 'NONE', *, *, #12754, .T. ) ;
#3094=CARTESIAN_POINT ( 'NONE',  ( -15.50000000000000000, -2.500000000000000000, 23.94337567297399971 ) ) ;
#3097=VERTEX_POINT ( 'NONE', #7894 ) ;
#3106=CYLINDRICAL_SURFACE ( 'NONE', #3606, 3.499999999999999556 ) ;
#3116=VERTEX_POINT ( 'NONE', #2939 ) ;
#3118=ORIENTED_EDGE ( 'NONE', *, *, #11866, .F. ) ;
#3122=CIRCLE ( 'NONE', #11786, 0.2000000000005226763 ) ;
#3137=ORIENTED_EDGE ( 'NONE', *, *, #3174, .T. ) ;
#3168=FACE_OUTER_BOUND ( 'NONE', #3259, .T. ) ;
#3170=ADVANCED_FACE ( 'NONE', ( #4329 ), #11460, .F. ) ;
#3174=EDGE_CURVE ( 'NONE', #51, #4925, #1695, .T. ) ;
#3192=DIRECTION ( 'NONE',  ( 0.000000000000000000, 1.000000000000000000, 0.000000000000000000 ) ) ;
#3198=DIRECTION ( 'NONE',  ( 0.000000000000000000, 0.000000000000000000, -1.000000000000000000 ) ) ;
#3200=EDGE_CURVE ( 'NONE', #11913, #9286, #4101, .T. ) ;
#3207=ORIENTED_EDGE ( 'NONE', *, *, #5948, .F. ) ;
#3222=( LENGTH_UNIT ( ) NAMED_UNIT ( * ) SI_UNIT ( .MILLI., .METRE. ) );
#3252=DIRECTION ( 'NONE',  ( 0.000000000000000000, 1.000000000000000000, 0.000000000000000000 ) ) ;
#3259=EDGE_LOOP ( 'NONE', ( #9270, #10468, #12809, #130 ) ) ;
#3265=EDGE_CURVE ( 'NONE', #777, #10300, #3568, .T. ) ;
#3274=FACE_OUTER_BOUND ( 'NONE', #2121, .T. ) ;
#3283=ORIENTED_EDGE ( 'NONE', *, *, #13299, .F. ) ;
#3292=AXIS2_PLACEMENT_3D ( 'NONE', #12543, #2925, #9967 ) ;
#3293=CARTESIAN_POINT ( 'NONE',  ( 14.25000000000000000, -0.2038245569916330158, -23.22168783648699986 ) ) ;
#3301=( NAMED_UNIT ( * ) SI_UNIT ( $, .STERADIAN. ) SOLID_ANGLE_UNIT ( ) );
#3316=AXIS2_PLACEMENT_3D ( 'NONE', #13432, #7622, #7547 ) ;
#3322=EDGE_LOOP ( 'NONE', ( #4478, #12052, #6178, #5192 ) ) ;
#3324=DIRECTION ( 'NONE',  ( 0.000000000000000000, 1.000000000000000000, 0.000000000000000000 ) ) ;
#3329=DIRECTION ( 'NONE',  ( 0.000000000000000000, 1.000000000000000000, 0.000000000000000000 ) ) ;
#3334=CARTESIAN_POINT ( 'NONE',  ( 15.50000000000000000, -0.2038245569916604938, -21.05662432702600029 ) ) ;
#3341=EDGE_LOOP ( 'NONE', ( #12495, #9657, #5611, #7391 ) ) ;
#3346=SURFACE_STYLE_FILL_AREA ( #13973 ) ;
#3350=CARTESIAN_POINT ( 'NONE',  ( 15.50000000000000000, -1.037157890325000054, 22.50000000000000000 ) ) ;
#3353=CARTESIAN_POINT ( 'NONE',  ( -14.25000000000000000, -2.500000000000000000, 21.77831216351300014 ) ) ;
#3355=B_SPLINE_CURVE_WITH_KNOTS ( 'NONE', 3,
 ( #932, #1166, #4433, #11640, #10546, #5691 ),
 .UNSPECIFIED., .F., .F.,
 ( 4, 2, 4 ),
 ( 0.0002380763768115301549, 0.7291065797294569162, 1.457975083082102330 ),
 .UNSPECIFIED. ) ;
#3361=ORIENTED_EDGE ( 'NONE', *, *, #580, .F. ) ;
#3371=DIRECTION ( 'NONE',  ( 0.000000000000000000, 0.000000000000000000, 1.000000000000000000 ) ) ;
#3373=CARTESIAN_POINT ( 'NONE',  ( 15.50000000000000000, -0.1999999999999999556, 22.50000000000000000 ) ) ;
#3378=ORIENTED_EDGE ( 'NONE', *, *, #6444, .T. ) ;
#3381=DIRECTION ( 'NONE',  ( 0.000000000000000000, 0.000000000000000000, 1.000000000000000000 ) ) ;
#3384=CARTESIAN_POINT ( 'NONE',  ( -14.66242688423474227, -0.3152598339554810170, 21.54019739087905094 ) ) ;
#3386=ORIENTED_EDGE ( 'NONE', *, *, #9660, .F. ) ;
#3417=ORIENTED_EDGE ( 'NONE', *, *, #9660, .T. ) ;
#3423=CARTESIAN_POINT ( 'NONE',  ( 0.000000000000000000, 0.000000000000000000, 0.000000000000000000 ) ) ;
#3438=DIRECTION ( 'NONE',  ( -1.000000000000000000, 0.000000000000000000, 0.000000000000000000 ) ) ;
#3441=ORIENTED_EDGE ( 'NONE', *, *, #13981, .T. ) ;
#3450=ORIENTED_EDGE ( 'NONE', *, *, #9487, .F. ) ;
#3451=CARTESIAN_POINT ( 'NONE',  ( 15.50000000000000000, -2.500000000000000000, 21.05662432702600029 ) ) ;
#3453=EDGE_CURVE ( 'NONE', #12945, #1628, #4872, .T. ) ;
#3459=EDGE_CURVE ( 'NONE', #13870, #14415, #7068, .T. ) ;
#3462=PLANE ( 'NONE',  #2156 ) ;
#3466=DIRECTION ( 'NONE',  ( -0.8660254037844482555, 0.000000000000000000, -0.4999999999999831801 ) ) ;
#3468=LINE ( 'NONE', #12864, #11195 ) ;
#3475=ORIENTED_EDGE ( 'NONE', *, *, #11238, .T. ) ;
#3485=CARTESIAN_POINT ( 'NONE',  ( 15.50000000000000000, -2.500000000000000000, 21.05662432702600029 ) ) ;
#3489=ORIENTED_EDGE ( 'NONE', *, *, #11200, .F. ) ;
#3496=DIRECTION ( 'NONE',  ( 0.000000000000000000, 0.000000000000000000, 1.000000000000000000 ) ) ;
#3499=CARTESIAN_POINT ( 'NONE',  ( -14.24999999999999822, -0.2715193793361453389, 22.98718409945082541 ) ) ;
#3500=PLANE ( 'NONE',  #7107 ) ;
#3504=DIRECTION ( 'NONE',  ( 0.000000000000000000, 0.000000000000000000, 1.000000000000000000 ) ) ;
#3509=CIRCLE ( 'NONE', #15143, 3.499999999999999556 ) ;
#3511=VERTEX_POINT ( 'NONE', #7433 ) ;
#3514=VECTOR ( 'NONE', #4745, 1000.000000000000000 ) ;
#3523=MECHANICAL_DESIGN_GEOMETRIC_PRESENTATION_REPRESENTATION('',(#11956),#11209);
#3525=ORIENTED_EDGE ( 'NONE', *, *, #6710, .T. ) ;
#3529=VECTOR ( 'NONE', #5143, 1000.000000000000114 ) ;
#3542=LINE ( 'NONE', #11618, #10711 ) ;
#3545=DIRECTION ( 'NONE',  ( 0.000000000000000000, 0.000000000000000000, 1.000000000000000000 ) ) ;
#3549=ORIENTED_EDGE ( 'NONE', *, *, #5714, .F. ) ;
#3554=AXIS2_PLACEMENT_3D ( 'NONE', #9130, #11693, #1059 ) ;
#3557=ADVANCED_FACE ( 'NONE', ( #14547 ), #356, .F. ) ;
#3562=EDGE_CURVE ( 'NONE', #10261, #6610, #11423, .T. ) ;
#3568=CIRCLE ( 'NONE', #1094, 1.449999999999999956 ) ;
#3570=ADVANCED_FACE ( 'NONE', ( #11582 ), #6713, .T. ) ;
#3578=CLOSED_SHELL ( 'NONE', ( #5437, #13207, #14077, #11920, #13533, #6618, #15206, #9409, #4234, #3170, #13609, #3744, #1479, #6595, #2524 ) ) ;
#3581=AXIS2_PLACEMENT_3D ( 'NONE', #13836, #4447, #868 ) ;
#3593=CARTESIAN_POINT ( 'NONE',  ( -15.50000000000000000, -2.500000000000000000, -23.94337567297399971 ) ) ;
#3603=VECTOR ( 'NONE', #11374, 1000.000000000000000 ) ;
#3604=CARTESIAN_POINT ( 'NONE',  ( -15.91242688423473517, -0.3152598339554900653, 21.29473909965994594 ) ) ;
#3605=DIRECTION ( 'NONE',  ( 0.000000000000000000, 1.000000000000000000, 0.000000000000000000 ) ) ;
#3606=AXIS2_PLACEMENT_3D ( 'NONE', #13657, #761, #1782 ) ;
#3613=AXIS2_PLACEMENT_3D ( 'NONE', #8399, #2656, #1495 ) ;
#3645=CARTESIAN_POINT ( 'NONE',  ( -16.75000000000000000, -2.500000000000000000, 23.22168783648699986 ) ) ;
#3651=EDGE_CURVE ( 'NONE', #7228, #3097, #15058, .T. ) ;
#3660=EDGE_CURVE ( 'NONE', #1915, #14331, #14617, .T. ) ;
#3665=CARTESIAN_POINT ( 'NONE',  ( 14.25000000000000000, -2.500000000000000000, -23.22168783648699986 ) ) ;
#3679=ORIENTED_EDGE ( 'NONE', *, *, #13981, .F. ) ;
#3681=CARTESIAN_POINT ( 'NONE',  ( -16.75000000000000000, -0.2038245569916330158, 21.77831216351300014 ) ) ;
#3696=CARTESIAN_POINT ( 'NONE',  ( -15.50000000000000000, -0.4000000000000000222, 22.50000000000000000 ) ) ;
#3702=VERTEX_POINT ( 'NONE', #13476 ) ;
#3717=ADVANCED_FACE ( 'NONE', ( #14901 ), #11021, .T. ) ;
#3719=DIRECTION ( 'NONE',  ( 0.000000000000000000, 0.000000000000000000, 1.000000000000000000 ) ) ;
#3727=CARTESIAN_POINT ( 'NONE',  ( -15.50000000000000000, -0.4000000000005236034, 19.20000000000052509 ) ) ;
#3730=DIRECTION ( 'NONE',  ( -0.8660254037844482555, 0.000000000000000000, -0.4999999999999831801 ) ) ;
#3739=ORIENTED_EDGE ( 'NONE', *, *, #805, .T. ) ;
#3742=ORIENTED_EDGE ( 'NONE', *, *, #15169, .F. ) ;
#3744=ADVANCED_FACE ( 'NONE', ( #1418, #2344 ), #11887, .T. ) ;
#3747=CARTESIAN_POINT ( 'NONE',  ( -16.75000000000000355, -0.2715193793361450614, -22.98718409945082541 ) ) ;
#3752=CYLINDRICAL_SURFACE ( 'NONE', #1635, 4.000000000000000000 ) ;
#3760=DIRECTION ( 'NONE',  ( 0.000000000000000000, 0.000000000000000000, 1.000000000000000000 ) ) ;
#3764=ORIENTED_EDGE ( 'NONE', *, *, #8205, .F. ) ;
#3768=AXIS2_PLACEMENT_3D ( 'NONE', #9585, #8659, #14323 ) ;
#3794=DIRECTION ( 'NONE',  ( 0.000000000000000000, 0.000000000000000000, 1.000000000000000000 ) ) ;
#3795=CARTESIAN_POINT ( 'NONE',  ( -14.24999999999999822, -0.2715193793361436736, -22.01281590054916038 ) ) ;
#3797=DIRECTION ( 'NONE',  ( 1.000000000000000000, 0.000000000000000000, 0.000000000000000000 ) ) ;
#3807=LINE ( 'NONE', #2646, #6803 ) ;
#3810=DIRECTION ( 'NONE',  ( -1.000000000000000000, 0.000000000000000000, 0.000000000000000000 ) ) ;
#3821=CARTESIAN_POINT ( 'NONE',  ( -15.50000000000000000, -1.037157890325000054, 22.50000000000000000 ) ) ;
#3822=VERTEX_POINT ( 'NONE', #7239 ) ;
#3829=AXIS2_PLACEMENT_3D ( 'NONE', #8438, #13184, #13035 ) ;
#3837=DIRECTION ( 'NONE',  ( 0.000000000000000000, 0.000000000000000000, 1.000000000000000000 ) ) ;
#3838=DIRECTION ( 'NONE',  ( 0.8660254037844482555, 0.000000000000000000, 0.4999999999999831801 ) ) ;
#3842=DIRECTION ( 'NONE',  ( 0.000000000000000000, 0.000000000000000000, 1.000000000000000000 ) ) ;
#3843=EDGE_CURVE ( 'NONE', #9156, #1855, #7319, .T. ) ;
#3859=CARTESIAN_POINT ( 'NONE',  ( -30.00000000000000000, -5.000000000000000000, -43.00000000000002132 ) ) ;
#3867=ADVANCED_BREP_SHAPE_REPRESENTATION ( '', ( #330, #298, #5426, #10531, #10636, #285 ), #14401 ) ;
#3874=AXIS2_PLACEMENT_3D ( 'NONE', #3373, #13849, #11441 ) ;
#3882=VECTOR ( 'NONE', #4392, 1000.000000000000114 ) ;
#3883=ORIENTED_EDGE ( 'NONE', *, *, #8478, .T. ) ;
#3899=DIRECTION ( 'NONE',  ( 0.000000000000000000, 1.000000000000000000, 0.000000000000000000 ) ) ;
#3904=UNCERTAINTY_MEASURE_WITH_UNIT (LENGTH_MEASURE( 1.000000000000000082E-05 ), #13130, 'distance_accuracy_value', 'NONE');
#3938=VERTEX_POINT ( 'NONE', #481 ) ;
#3939=VERTEX_POINT ( 'NONE', #6466 ) ;
#3944=VERTEX_POINT ( 'NONE', #14664 ) ;
#3955=CARTESIAN_POINT ( 'NONE',  ( 15.91434062215688350, -0.3156604612129282894, -23.70415600323552852 ) ) ;
#3960=ORIENTED_EDGE ( 'NONE', *, *, #3200, .T. ) ;
#3961=LINE ( 'NONE', #1779, #2334 ) ;
#3973=VERTEX_POINT ( 'NONE', #12354 ) ;
#3983=DIRECTION ( 'NONE',  ( 0.000000000000000000, 0.000000000000000000, 1.000000000000000000 ) ) ;
#3984=EDGE_CURVE ( 'NONE', #5926, #7246, #240, .T. ) ;
#3998=CARTESIAN_POINT ( 'NONE',  ( 15.50000000000000000, -5.000000000000000000, 22.50000000000000000 ) ) ;
#4001=AXIS2_PLACEMENT_3D ( 'NONE', #960, #5713, #7944 ) ;
#4004=LINE ( 'NONE', #12319, #13546 ) ;
#4015=DIRECTION ( 'NONE',  ( 0.000000000000000000, 1.000000000000000000, 0.000000000000000000 ) ) ;
#4017=VECTOR ( 'NONE', #860, 1000.000000000000000 ) ;
#4027=ORIENTED_EDGE ( 'NONE', *, *, #12466, .F. ) ;
#4028=CARTESIAN_POINT ( 'NONE',  ( 14.05000000000000249, -0.2000000000000000111, -22.50000000000000000 ) ) ;
#4036=ORIENTED_EDGE ( 'NONE', *, *, #11866, .T. ) ;
#4037=DIRECTION ( 'NONE',  ( 0.000000000000000000, 0.000000000000000000, 1.000000000000000000 ) ) ;
#4041=DIRECTION ( 'NONE',  ( 0.000000000000000000, 1.000000000000000000, 0.000000000000000000 ) ) ;
#4045=ADVANCED_FACE ( 'NONE', ( #11564 ), #15040, .T. ) ;
#4076=EDGE_LOOP ( 'NONE', ( #12161, #7975, #10642, #15115 ) ) ;
#4078=ORIENTED_EDGE ( 'NONE', *, *, #14917, .T. ) ;
#4084=DIRECTION ( 'NONE',  ( 0.000000000000000000, 0.000000000000000000, 1.000000000000000000 ) ) ;
#4086=DIRECTION ( 'NONE',  ( -1.000000000000000000, 0.000000000000000000, 0.000000000000000000 ) ) ;
#4088=DIRECTION ( 'NONE',  ( 0.000000000000000000, 0.000000000000000000, -1.000000000000000000 ) ) ;
#4097=EDGE_CURVE ( 'NONE', #5891, #8137, #6841, .T. ) ;
#4101=LINE ( 'NONE', #14790, #2076 ) ;
#4104=DIRECTION ( 'NONE',  ( 0.000000000000000000, 1.000000000000000000, 0.000000000000000000 ) ) ;
#4105=AXIS2_PLACEMENT_3D ( 'NONE', #12170, #13420, #12105 ) ;
#4107=DIRECTION ( 'NONE',  ( 1.060575238724893480E-16, 0.5000000000000189848, -0.8660254037844277164 ) ) ;
#4118=AXIS2_PLACEMENT_3D ( 'NONE', #11830, #13228, #15304 ) ;
#4120=AXIS2_PLACEMENT_3D ( 'NONE', #2926, #7736, #4086 ) ;
#4132=AXIS2_PLACEMENT_3D ( 'NONE', #14128, #14507, #12044 ) ;
#4136=EDGE_CURVE ( 'NONE', #5494, #14030, #12722, .T. ) ;
#4141=LINE ( 'NONE', #11272, #5502 ) ;
#4148=CARTESIAN_POINT ( 'NONE',  ( 14.25000000000000000, -0.2038245569916330158, -23.22168783648699986 ) ) ;
#4153=EDGE_LOOP ( 'NONE', ( #13314, #1852, #1423, #11744 ) ) ;
#4172=ORIENTED_EDGE ( 'NONE', *, *, #10258, .F. ) ;
#4173=VECTOR ( 'NONE', #4661, 1000.000000000000000 ) ;
#4177=FACE_BOUND ( 'NONE', #11802, .T. ) ;
#4181=CARTESIAN_POINT ( 'NONE',  ( -15.50000000000000000, 998.9628421096749662, -22.50000000000000000 ) ) ;
#4182=DIRECTION ( 'NONE',  ( 0.4999999999999827360, 0.000000000000000000, 0.8660254037844485886 ) ) ;
#4186=EDGE_LOOP ( 'NONE', ( #7973, #3960, #7484, #2458 ) ) ;
#4189=ORIENTED_EDGE ( 'NONE', *, *, #10652, .F. ) ;
#4192=EDGE_LOOP ( 'NONE', ( #1109, #1254, #3475, #8246 ) ) ;
#4203=FACE_OUTER_BOUND ( 'NONE', #12173, .T. ) ;
#4204=EDGE_CURVE ( 'NONE', #14751, #8552, #11023, .T. ) ;
#4205=CARTESIAN_POINT ( 'NONE',  ( 16.75000000000000000, -0.2038245569916320166, 23.22168783648699986 ) ) ;
#4223=CARTESIAN_POINT ( 'NONE',  ( 15.08565937784311117, -0.3156604612129225162, 23.70415600323552852 ) ) ;
#4226=ORIENTED_EDGE ( 'NONE', *, *, #13577, .F. ) ;
#4229=VERTEX_POINT ( 'NONE', #2241 ) ;
#4234=ADVANCED_FACE ( 'NONE', ( #14187 ), #2471, .F. ) ;
#4240=CARTESIAN_POINT ( 'NONE',  ( 16.75000000000000000, -2.500000000000000000, 23.22168783648699986 ) ) ;
#4254=CARTESIAN_POINT ( 'NONE',  ( -14.66434062215825840, -0.3156604612126666654, 23.46090750622624910 ) ) ;
#4273=CARTESIAN_POINT ( 'NONE',  ( -16.75000000000000000, -0.2038245569916330158, -21.77831216351300014 ) ) ;
#4275=VERTEX_POINT ( 'NONE', #5756 ) ;
#4278=ORIENTED_EDGE ( 'NONE', *, *, #3660, .T. ) ;
#4283=PLANE ( 'NONE',  #10705 ) ;
#4287=VECTOR ( 'NONE', #7981, 1000.000000000000000 ) ;
#4292=DIRECTION ( 'NONE',  ( 0.8660254037844482555, 0.000000000000000000, -0.4999999999999831801 ) ) ;
#4306=DIRECTION ( 'NONE',  ( 0.000000000000000000, 0.000000000000000000, 1.000000000000000000 ) ) ;
#4307=CARTESIAN_POINT ( 'NONE',  ( 15.50000000000000000, -0.4000000000005274892, 22.50000000000000000 ) ) ;
#4313=EDGE_CURVE ( 'NONE', #8137, #1184, #3122, .T. ) ;
#4316=CARTESIAN_POINT ( 'NONE',  ( 15.50000000000000000, -0.2000000000000000111, 22.50000000000000000 ) ) ;
#4318=VERTEX_POINT ( 'NONE', #2709 ) ;
#4323=CONICAL_SURFACE ( 'NONE', #3316, 1732.050807568785558, 1.047197551196574761 ) ;
#4324=AXIS2_PLACEMENT_3D ( 'NONE', #12227, #13101, #9581 ) ;
#4329=FACE_OUTER_BOUND ( 'NONE', #8432, .T. ) ;
#4334=DIRECTION ( 'NONE',  ( 0.000000000000000000, 1.000000000000000000, 0.000000000000000000 ) ) ;
#4336=AXIS2_PLACEMENT_3D ( 'NONE', #9378, #8381, #5919 ) ;
#4359=ORIENTED_EDGE ( 'NONE', *, *, #11240, .F. ) ;
#4370=CARTESIAN_POINT ( 'NONE',  ( 15.50000000000000000, -0.2038245569916610489, -23.94337567297399971 ) ) ;
#4374=ORIENTED_EDGE ( 'NONE', *, *, #10279, .T. ) ;
#4388=CIRCLE ( 'NONE', #6389, 4.000000000000000000 ) ;
#4389=EDGE_CURVE ( 'NONE', #10402, #51, #13024, .T. ) ;
#4392=DIRECTION ( 'NONE',  ( 0.8660254037844482555, 0.000000000000000000, -0.4999999999999831801 ) ) ;
#4395=FILL_AREA_STYLE_COLOUR ( '', #5843 ) ;
#4399=ADVANCED_FACE ( 'NONE', ( #531 ), #5354, .T. ) ;
#4403=EDGE_CURVE ( 'NONE', #4486, #2946, #12021, .T. ) ;
#4433=CARTESIAN_POINT ( 'NONE',  ( -14.66242688423474227, -0.3152598339554795182, -23.45980260912095616 ) ) ;
#4435=AXIS2_PLACEMENT_3D ( 'NONE', #14697, #12085, #4084 ) ;
#4436=VERTEX_POINT ( 'NONE', #7533 ) ;
#4437=ORIENTED_EDGE ( 'NONE', *, *, #2625, .T. ) ;
#4445=CARTESIAN_POINT ( 'NONE',  ( -15.50000000000000000, -2.500000000000000000, -23.94337567297399971 ) ) ;
#4447=DIRECTION ( 'NONE',  ( 1.000000000000000000, 0.000000000000000000, 0.000000000000000000 ) ) ;
#4458=CARTESIAN_POINT ( 'NONE',  ( -15.50000000000000000, -5.000000000000000000, -22.50000000000000000 ) ) ;
#4465=ORIENTED_EDGE ( 'NONE', *, *, #6320, .F. ) ;
#4466=SURFACE_STYLE_USAGE ( .BOTH. , #10274 ) ;
#4469=ADVANCED_FACE ( 'NONE', ( #3014 ), #9127, .F. ) ;
#4474=CARTESIAN_POINT ( 'NONE',  ( -15.50000000000000000, -0.2000000000000000111, 25.79999999999947136 ) ) ;
#4478=ORIENTED_EDGE ( 'NONE', *, *, #9056, .F. ) ;
#4485=EDGE_CURVE ( 'NONE', #5494, #3511, #7756, .T. ) ;
#4486=VERTEX_POINT ( 'NONE', #1844 ) ;
#4510=ADVANCED_FACE ( 'NONE', ( #907 ), #7827, .F. ) ;
#4515=EDGE_CURVE ( 'NONE', #5656, #1184, #14752, .T. ) ;
#4522=CARTESIAN_POINT ( 'NONE',  ( -15.50000000000000000, -2.500000000000000000, -21.05662432702600029 ) ) ;
#4528=ORIENTED_EDGE ( 'NONE', *, *, #1070, .F. ) ;
#4534=CARTESIAN_POINT ( 'NONE',  ( 15.50000000000000000, -5.000000000000000000, -18.50000000000000000 ) ) ;
#4535=CARTESIAN_POINT ( 'NONE',  ( 15.50000000000000000, -5.000000000000000000, 19.00000000000000000 ) ) ;
#4544=VECTOR ( 'NONE', #3797, 1000.000000000000000 ) ;
#4551=AXIS2_PLACEMENT_3D ( 'NONE', #7900, #15167, #4559 ) ;
#4552=DIRECTION ( 'NONE',  ( 0.000000000000000000, 0.000000000000000000, 1.000000000000000000 ) ) ;
#4559=DIRECTION ( 'NONE',  ( 0.000000000000000000, 0.000000000000000000, 1.000000000000000000 ) ) ;
#4572=DIRECTION ( 'NONE',  ( 0.8660254037844482555, 0.000000000000000000, 0.4999999999999831801 ) ) ;
#4574=DIRECTION ( 'NONE',  ( 0.000000000000000000, 1.000000000000000000, 0.000000000000000000 ) ) ;
#4581=ORIENTED_EDGE ( 'NONE', *, *, #12297, .T. ) ;
#4586=MECHANICAL_DESIGN_GEOMETRIC_PRESENTATION_REPRESENTATION('',(#10058),#6586);
#4597=( GEOMETRIC_REPRESENTATION_CONTEXT ( 3 ) GLOBAL_UNCERTAINTY_ASSIGNED_CONTEXT ( ( #15048 ) ) GLOBAL_UNIT_ASSIGNED_CONTEXT ( ( #3222, #10425, #3301 ) ) REPRESENTATION_CONTEXT ( 'NONE', 'WORKASPACE' ) );
#4607=EDGE_CURVE ( 'NONE', #10402, #3944, #4716, .T. ) ;
#4608=VERTEX_POINT ( 'NONE', #4792 ) ;
#4609=EDGE_LOOP ( 'NONE', ( #8625, #6214, #3742, #7340 ) ) ;
#4614=CIRCLE ( 'NONE', #3874, 1.449999999999996403 ) ;
#4619=DIRECTION ( 'NONE',  ( 0.000000000000000000, 1.000000000000000000, 0.000000000000000000 ) ) ;
#4627=VECTOR ( 'NONE', #7864, 1000.000000000000000 ) ;
#4631=( LENGTH_UNIT ( ) NAMED_UNIT ( * ) SI_UNIT ( .MILLI., .METRE. ) );
#4639=DIRECTION ( 'NONE',  ( 0.000000000000000000, 1.000000000000000000, 0.000000000000000000 ) ) ;
#4647=ORIENTED_EDGE ( 'NONE', *, *, #12754, .F. ) ;
#4652=ORIENTED_EDGE ( 'NONE', *, *, #9056, .T. ) ;
#4658=EDGE_CURVE ( 'NONE', #13129, #5656, #5601, .T. ) ;
#4661=DIRECTION ( 'NONE',  ( -1.284980352575412699E-16, -0.000000000000000000, -1.000000000000000000 ) ) ;
#4688=VERTEX_POINT ( 'NONE', #7049 ) ;
#4689=EDGE_LOOP ( 'NONE', ( #9003, #10685, #7081, #2947 ) ) ;
#4716=LINE ( 'NONE', #12863, #8059 ) ;
#4720=VERTEX_POINT ( 'NONE', #1684 ) ;
#4723=ORIENTED_EDGE ( 'NONE', *, *, #6528, .F. ) ;
#4738=EDGE_LOOP ( 'NONE', ( #2916, #13198 ) ) ;
#4745=DIRECTION ( 'NONE',  ( 0.000000000000000000, 1.000000000000000000, 0.000000000000000000 ) ) ;
#4750=LINE ( 'NONE', #1102, #833 ) ;
#4761=CARTESIAN_POINT ( 'NONE',  ( -16.75000000000000000, -0.3156864504677179273, -22.74361999681790536 ) ) ;
#4765=ORIENTED_EDGE ( 'NONE', *, *, #9772, .T. ) ;
#4774=EDGE_CURVE ( 'NONE', #6230, #4906, #15246, .T. ) ;
#4780=EDGE_LOOP ( 'NONE', ( #15062, #5617, #11700, #4528 ) ) ;
#4792=CARTESIAN_POINT ( 'NONE',  ( -15.50000000000000000, -5.000000000000000000, -26.50000000000000000 ) ) ;
#4794=VECTOR ( 'NONE', #7853, 1000.000000000000000 ) ;
#4798=EDGE_CURVE ( 'NONE', #6810, #1528, #4004, .T. ) ;
#4800=EDGE_CURVE ( 'NONE', #2099, #9156, #8589, .T. ) ;
#4812=LINE ( 'NONE', #14186, #4173 ) ;
#4813=SURFACE_STYLE_USAGE ( .BOTH. , #7532 ) ;
#4832=CARTESIAN_POINT ( 'NONE',  ( -16.75000000000000000, -2.500000000000000000, -21.77831216351300014 ) ) ;
#4833=DIRECTION ( 'NONE',  ( 0.000000000000000000, 1.000000000000000000, 0.000000000000000000 ) ) ;
#4872=LINE ( 'NONE', #1368, #5577 ) ;
#4876=PLANE ( 'NONE',  #2796 ) ;
#4886=ORIENTED_EDGE ( 'NONE', *, *, #11424, .F. ) ;
#4894=ADVANCED_FACE ( 'NONE', ( #9968 ), #512, .T. ) ;
#4901=CARTESIAN_POINT ( 'NONE',  ( -15.50000000000000000, -1.037157890325000054, 22.50000000000000000 ) ) ;
#4902=ORIENTED_EDGE ( 'NONE', *, *, #2519, .T. ) ;
#4905=EDGE_CURVE ( 'NONE', #14839, #3822, #8892, .T. ) ;
#4906=VERTEX_POINT ( 'NONE', #10045 ) ;
#4914=LINE ( 'NONE', #3665, #11306 ) ;
#4918=CARTESIAN_POINT ( 'NONE',  ( 14.05000000000000249, -0.2000000000000000111, 22.50000000000000000 ) ) ;
#4925=VERTEX_POINT ( 'NONE', #7884 ) ;
#4929=DIRECTION ( 'NONE',  ( 0.000000000000000000, 1.000000000000000000, 0.000000000000000000 ) ) ;
#4951=EDGE_CURVE ( 'NONE', #7246, #14906, #2877, .T. ) ;
#4980=EDGE_CURVE ( 'NONE', #13163, #11286, #6581, .T. ) ;
#4986=CARTESIAN_POINT ( 'NONE',  ( 15.50000000000000000, -1.037157890325000054, -22.50000000000000000 ) ) ;
#4994=ADVANCED_FACE ( 'NONE', ( #6477 ), #3752, .F. ) ;
#5000=DIRECTION ( 'NONE',  ( 0.000000000000000000, 1.000000000000000000, 0.000000000000000000 ) ) ;
#5001=DIRECTION ( 'NONE',  ( 0.000000000000000000, 1.000000000000000000, 0.000000000000000000 ) ) ;
#5008=TOROIDAL_SURFACE ( 'NONE', #13678, 3.299999999999474909, 0.2000000000005234813 ) ;
#5013=EDGE_LOOP ( 'NONE', ( #6748, #8591 ) ) ;
#5024=AXIS2_PLACEMENT_3D ( 'NONE', #2136, #5797, #10503 ) ;
#5027=EDGE_LOOP ( 'NONE', ( #14176, #14800, #13505, #14398 ) ) ;
#5032=EDGE_LOOP ( 'NONE', ( #7719, #10524, #5905, #12636 ) ) ;
#5041=CARTESIAN_POINT ( 'NONE',  ( 14.66242688423474050, -0.3152598339554796292, -21.54019739087904384 ) ) ;
#5042=EDGE_CURVE ( 'NONE', #181, #4720, #13457, .T. ) ;
#5043=CARTESIAN_POINT ( 'NONE',  ( -30.00000000000000000, -5.000000000000000000, 27.00000000000000000 ) ) ;
#5044=EDGE_LOOP ( 'NONE', ( #12380, #6589 ) ) ;
#5046=AXIS2_PLACEMENT_3D ( 'NONE', #4307, #8024, #9034 ) ;
#5048=ORIENTED_EDGE ( 'NONE', *, *, #2193, .F. ) ;
#5053=DIRECTION ( 'NONE',  ( -1.000000000000000000, 0.000000000000000000, 0.000000000000000000 ) ) ;
#5069=ORIENTED_EDGE ( 'NONE', *, *, #2419, .T. ) ;
#5074=EDGE_CURVE ( 'NONE', #6450, #4436, #5078, .T. ) ;
#5078=LINE ( 'NONE', #9870, #408 ) ;
#5102=CARTESIAN_POINT ( 'NONE',  ( 15.50000000000000000, -0.2038245569916604938, 23.94337567297399971 ) ) ;
#5109=DIRECTION ( 'NONE',  ( 0.000000000000000000, 1.000000000000000000, 0.000000000000000000 ) ) ;
#5130=DIRECTION ( 'NONE',  ( 0.000000000000000000, 1.000000000000000000, 0.000000000000000000 ) ) ;
#5132=ORIENTED_EDGE ( 'NONE', *, *, #4980, .T. ) ;
#5143=DIRECTION ( 'NONE',  ( 0.8660254037844482555, 0.000000000000000000, 0.4999999999999831801 ) ) ;
#5147=CARTESIAN_POINT ( 'NONE',  ( 15.50000000000000000, -5.000000000000000000, -26.00000000000000000 ) ) ;
#5149=CYLINDRICAL_SURFACE ( 'NONE', #10737, 4.000000000000000000 ) ;
#5161=CARTESIAN_POINT ( 'NONE',  ( 16.75000000000000000, -2.500000000000000000, 23.22168783648699986 ) ) ;
#5163=LINE ( 'NONE', #9872, #8340 ) ;
#5165=FACE_OUTER_BOUND ( 'NONE', #4738, .T. ) ;
#5169=CARTESIAN_POINT ( 'NONE',  ( 14.25000000000000000, -2.500000000000000000, -23.22168783648699986 ) ) ;
#5171=ORIENTED_EDGE ( 'NONE', *, *, #12867, .F. ) ;
#5184=CARTESIAN_POINT ( 'NONE',  ( -15.50000000000000000, -2.500000000000000000, 21.05662432702600029 ) ) ;
#5190=CARTESIAN_POINT ( 'NONE',  ( 15.50000000000000000, -1.037157890325000054, -22.50000000000000000 ) ) ;
#5192=ORIENTED_EDGE ( 'NONE', *, *, #4798, .F. ) ;
#5199=SURFACE_SIDE_STYLE ('',( #5504 ) ) ;
#5200=CARTESIAN_POINT ( 'NONE',  ( -14.25000000000000178, -0.2714405302574905976, -22.98746066354537732 ) ) ;
#5208=EDGE_LOOP ( 'NONE', ( #37, #12469, #14824, #11249 ) ) ;
#5228=FACE_OUTER_BOUND ( 'NONE', #4076, .T. ) ;
#5248=DIRECTION ( 'NONE',  ( 0.000000000000000000, 1.000000000000000000, 0.000000000000000000 ) ) ;
#5249=PLANE ( 'NONE',  #3292 ) ;
#5266=CIRCLE ( 'NONE', #13185, 0.2000000000005226763 ) ;
#5272=( NAMED_UNIT ( * ) PLANE_ANGLE_UNIT ( ) SI_UNIT ( $, .RADIAN. ) );
#5275=CARTESIAN_POINT ( 'NONE',  ( -15.50000000000000000, -1.037157890325000054, 22.50000000000000000 ) ) ;
#5279=CARTESIAN_POINT ( 'NONE',  ( -14.25000000000000000, -0.2038245569916330158, 23.22168783648699986 ) ) ;
#5285=ORIENTED_EDGE ( 'NONE', *, *, #6219, .F. ) ;
#5287=EDGE_CURVE ( 'NONE', #9156, #12927, #13861, .T. ) ;
#5298=TOROIDAL_SURFACE ( 'NONE', #5046, 3.299999999999470024, 0.2000000000005275058 ) ;
#5299=DIRECTION ( 'NONE',  ( 0.000000000000000000, 0.000000000000000000, -1.000000000000000000 ) ) ;
#5317=EDGE_LOOP ( 'NONE', ( #12865, #8389, #13803, #7762 ) ) ;
#5335=EDGE_LOOP ( 'NONE', ( #5672, #1669, #3764, #363 ) ) ;
#5345=PRODUCT ( 'Mounting Plate', 'Mounting Plate', '', ( #7033 ) ) ;
#5346=EDGE_CURVE ( 'NONE', #3973, #9206, #5894, .T. ) ;
#5349=CLOSED_SHELL ( 'NONE', ( #4045, #6235, #8484, #12288, #14557, #9697, #5563, #2712, #12860, #5869, #12148, #11906, #7809, #12832, #10835 ) ) ;
#5353=DIRECTION ( 'NONE',  ( 0.8660254037844482555, 0.000000000000000000, 0.4999999999999831801 ) ) ;
#5354=TOROIDAL_SURFACE ( 'NONE', #4105, 3.299999999999474909, 0.2000000000005234813 ) ;
#5366=AXIS2_PLACEMENT_3D ( 'NONE', #14223, #3605, #7257 ) ;
#5380=DIRECTION ( 'NONE',  ( 1.000000000000000000, 0.000000000000000000, 0.000000000000000000 ) ) ;
#5383=EDGE_CURVE ( 'NONE', #1528, #1551, #13557, .T. ) ;
#5389=EDGE_LOOP ( 'NONE', ( #7156, #4078, #8139, #9611 ) ) ;
#5391=CARTESIAN_POINT ( 'NONE',  ( 14.25000000000000000, -0.2038245569916330158, 23.22168783648699986 ) ) ;
#5395=AXIS2_PLACEMENT_3D ( 'NONE', #8376, #10778, #11706 ) ;
#5403=ORIENTED_EDGE ( 'NONE', *, *, #1095, .T. ) ;
#5410=ORIENTED_EDGE ( 'NONE', *, *, #3453, .T. ) ;
#5414=CARTESIAN_POINT ( 'NONE',  ( -16.75000000000000000, -2.500000000000000000, 21.77831216351300014 ) ) ;
#5424=ORIENTED_EDGE ( 'NONE', *, *, #8833, .F. ) ;
#5426=MANIFOLD_SOLID_BREP ( 'Cut-Extrude1[4]', #5349 ) ;
#5431=CARTESIAN_POINT ( 'NONE',  ( -15.50000000000000000, -0.1999999999999999556, -22.50000000000000000 ) ) ;
#5437=ADVANCED_FACE ( 'NONE', ( #7232 ), #7395, .T. ) ;
#5442=EDGE_LOOP ( 'NONE', ( #10273, #7971, #9666, #281 ) ) ;
#5448=CARTESIAN_POINT ( 'NONE',  ( 16.75000000000000000, -0.2038245569916320166, -23.22168783648699986 ) ) ;
#5459=ORIENTED_EDGE ( 'NONE', *, *, #2600, .F. ) ;
#5464=EDGE_CURVE ( 'NONE', #10251, #3023, #12026, .T. ) ;
#5466=CARTESIAN_POINT ( 'NONE',  ( -23.24999999999999289, -5.000000000000000000, -27.00000000000000000 ) ) ;
#5474=EDGE_CURVE ( 'NONE', #11913, #6450, #9619, .T. ) ;
#5477=CARTESIAN_POINT ( 'NONE',  ( -16.75000000000000000, -2.500000000000000000, 23.22168783648699986 ) ) ;
#5491=DIRECTION ( 'NONE',  ( 0.000000000000000000, 0.000000000000000000, -1.000000000000000000 ) ) ;
#5492=DIRECTION ( 'NONE',  ( 0.000000000000000000, 0.000000000000000000, 1.000000000000000000 ) ) ;
#5494=VERTEX_POINT ( 'NONE', #14875 ) ;
#5502=VECTOR ( 'NONE', #12435, 1000.000000000000000 ) ;
#5504=SURFACE_STYLE_FILL_AREA ( #7755 ) ;
#5505=DIRECTION ( 'NONE',  ( 0.000000000000000000, 0.000000000000000000, 1.000000000000000000 ) ) ;
#5508=EDGE_LOOP ( 'NONE', ( #14006, #2017, #3489, #15045, #6472, #9118 ) ) ;
#5509=DIRECTION ( 'NONE',  ( 0.4999999999999827360, 0.000000000000000000, -0.8660254037844485886 ) ) ;
#5511=VECTOR ( 'NONE', #6, 1000.000000000000000 ) ;
#5516=EDGE_LOOP ( 'NONE', ( #6364, #2717, #671, #6209 ) ) ;
#5523=CARTESIAN_POINT ( 'NONE',  ( 15.50000000000000000, -0.1999999999999999556, -21.05000000000000426 ) ) ;
#5527=CARTESIAN_POINT ( 'NONE',  ( 14.25000000000000000, -2.500000000000000000, -21.77831216351300014 ) ) ;
#5532=CONICAL_SURFACE ( 'NONE', #12209, 1732.050807568789651, 1.047197551196575871 ) ;
#5534=ORIENTED_EDGE ( 'NONE', *, *, #4905, .T. ) ;
#5553=ADVANCED_FACE ( 'NONE', ( #9072, #7909, #12640, #6460, #14734 ), #2879, .T. ) ;
#5562=CARTESIAN_POINT ( 'NONE',  ( -15.50000000000000000, -1.037157890325000054, -18.50000000000000000 ) ) ;
#5563=ADVANCED_FACE ( 'NONE', ( #544 ), #3106, .T. ) ;
#5564=PLANE ( 'NONE',  #12780 ) ;
#5568=DIRECTION ( 'NONE',  ( 0.000000000000000000, 0.000000000000000000, 1.000000000000000000 ) ) ;
#5576=VECTOR ( 'NONE', #14500, 1000.000000000000000 ) ;
#5577=VECTOR ( 'NONE', #7279, 1000.000000000000000 ) ;
#5582=CARTESIAN_POINT ( 'NONE',  ( 14.25000000000000000, -2.500000000000000000, 21.77831216351300014 ) ) ;
#5601=CIRCLE ( 'NONE', #2862, 0.2000000000005226763 ) ;
#5603=CARTESIAN_POINT ( 'NONE',  ( -31.00000000000000000, -2.500000000000000000, 0.000000000000000000 ) ) ;
#5611=ORIENTED_EDGE ( 'NONE', *, *, #2723, .T. ) ;
#5617=ORIENTED_EDGE ( 'NONE', *, *, #2505, .T. ) ;
#5624=CARTESIAN_POINT ( 'NONE',  ( -14.25000000000000000, -0.2038245569916330158, 21.77831216351300014 ) ) ;
#5628=FACE_OUTER_BOUND ( 'NONE', #8189, .T. ) ;
#5634=EDGE_LOOP ( 'NONE', ( #4902, #14368, #5459, #13616 ) ) ;
#5635=ORIENTED_EDGE ( 'NONE', *, *, #997, .T. ) ;
#5638=ORIENTED_EDGE ( 'NONE', *, *, #339, .F. ) ;
#5644=DIRECTION ( 'NONE',  ( 0.000000000000000000, 1.000000000000000000, 0.000000000000000000 ) ) ;
#5648=DIRECTION ( 'NONE',  ( 0.000000000000000000, 1.000000000000000000, 0.000000000000000000 ) ) ;
#5656=VERTEX_POINT ( 'NONE', #7353 ) ;
#5670=ORIENTED_EDGE ( 'NONE', *, *, #10272, .F. ) ;
#5672=ORIENTED_EDGE ( 'NONE', *, *, #5673, .T. ) ;
#5673=EDGE_CURVE ( 'NONE', #14751, #382, #10533, .T. ) ;
#5674=ORIENTED_EDGE ( 'NONE', *, *, #11826, .F. ) ;
#5683=CARTESIAN_POINT ( 'NONE',  ( -15.50000000000000000, 0.000000000000000000, -26.50000000000000000 ) ) ;
#5691=CARTESIAN_POINT ( 'NONE',  ( -15.50000000000000000, -0.2038245569916614930, -23.94337567297399971 ) ) ;
#5693=ORIENTED_EDGE ( 'NONE', *, *, #967, .T. ) ;
#5700=DIRECTION ( 'NONE',  ( 0.000000000000000000, 1.000000000000000000, 0.000000000000000000 ) ) ;
#5709=ORIENTED_EDGE ( 'NONE', *, *, #7727, .F. ) ;
#5713=DIRECTION ( 'NONE',  ( 1.000000000000000000, -0.000000000000000000, 1.224646799147353207E-16 ) ) ;
#5714=EDGE_CURVE ( 'NONE', #14910, #4229, #1211, .T. ) ;
#5722=VERTEX_POINT ( 'NONE', #5683 ) ;
#5725=ORIENTED_EDGE ( 'NONE', *, *, #7721, .F. ) ;
#5736=CARTESIAN_POINT ( 'NONE',  ( -14.25000000000000000, -2.500000000000000000, 21.77831216351300014 ) ) ;
#5748=EDGE_CURVE ( 'NONE', #11599, #1408, #13559, .T. ) ;
#5749=AXIS2_PLACEMENT_3D ( 'NONE', #10813, #178, #5867 ) ;
#5751=PLANE ( 'NONE',  #9225 ) ;
#5755=CARTESIAN_POINT ( 'NONE',  ( -15.50000000000000000, -0.2000000000000000111, 22.50000000000000000 ) ) ;
#5756=CARTESIAN_POINT ( 'NONE',  ( 15.50000000000000000, -2.500000000000000000, 23.94337567297399971 ) ) ;
#5764=ORIENTED_EDGE ( 'NONE', *, *, #10649, .F. ) ;
#5776=DIRECTION ( 'NONE',  ( 0.000000000000000000, 1.000000000000000000, 0.000000000000000000 ) ) ;
#5779=EDGE_LOOP ( 'NONE', ( #5285, #13278, #7012, #14158 ) ) ;
#5797=DIRECTION ( 'NONE',  ( 0.000000000000000000, 1.000000000000000000, 0.000000000000000000 ) ) ;
#5801=( NAMED_UNIT ( * ) SI_UNIT ( $, .STERADIAN. ) SOLID_ANGLE_UNIT ( ) );
#5809=DIRECTION ( 'NONE',  ( -0.000000000000000000, 1.000000000000000000, -0.000000000000000000 ) ) ;
#5825=VERTEX_POINT ( 'NONE', #6494 ) ;
#5841=ORIENTED_EDGE ( 'NONE', *, *, #14053, .F. ) ;
#5843=COLOUR_RGB ( '', 0.09019608, 0.27058824, 0.51372549) ;
#5853=DIRECTION ( 'NONE',  ( 0.000000000000000000, 0.000000000000000000, 1.000000000000000000 ) ) ;
#5855=CARTESIAN_POINT ( 'NONE',  ( 16.75000000000000000, -2.500000000000000000, -21.77831216351300014 ) ) ;
#5866=VERTEX_POINT ( 'NONE', #5102 ) ;
#5867=DIRECTION ( 'NONE',  ( 0.000000000000000000, 0.000000000000000000, 1.000000000000000000 ) ) ;
#5869=ADVANCED_FACE ( 'NONE', ( #12613 ), #9259, .F. ) ;
#5871=ADVANCED_FACE ( 'NONE', ( #1974 ), #5564, .F. ) ;
#5876=CONICAL_SURFACE ( 'NONE', #4118, 1732.050807568785558, 1.047197551196574761 ) ;
#5883=ORIENTED_EDGE ( 'NONE', *, *, #1810, .T. ) ;
#5884=AXIS2_PLACEMENT_3D ( 'NONE', #7777, #12510, #1717 ) ;
#5886=DIRECTION ( 'NONE',  ( 0.000000000000000000, 1.000000000000000000, 0.000000000000000000 ) ) ;
#5891=VERTEX_POINT ( 'NONE', #961 ) ;
#5894=B_SPLINE_CURVE_WITH_KNOTS ( 'NONE', 3,
 ( #6927, #2338, #12818, #13133, #7003, #12976 ),
 .UNSPECIFIED., .F., .F.,
 ( 4, 2, 4 ),
 ( 0.0002380763768130567115, 0.7291065797294590256, 1.457975083082104995 ),
 .UNSPECIFIED. ) ;
#5905=ORIENTED_EDGE ( 'NONE', *, *, #3200, .F. ) ;
#5913=CARTESIAN_POINT ( 'NONE',  ( -30.00000000000000000, -5.000000000000000000, -43.00000000000002132 ) ) ;
#5914=CARTESIAN_POINT ( 'NONE',  ( -16.75000000000000000, -2.500000000000000000, -21.77831216351300014 ) ) ;
#5915=ADVANCED_FACE ( 'NONE', ( #2130 ), #14514, .F. ) ;
#5919=DIRECTION ( 'NONE',  ( 0.000000000000000000, 0.000000000000000000, 1.000000000000000000 ) ) ;
#5925=EDGE_LOOP ( 'NONE', ( #12131, #8519, #3450, #7618 ) ) ;
#5926=VERTEX_POINT ( 'NONE', #4535 ) ;
#5928=AXIS2_PLACEMENT_3D ( 'NONE', #5755, #4574, #7913 ) ;
#5932=LINE ( 'NONE', #77, #3514 ) ;
#5935=CARTESIAN_POINT ( 'NONE',  ( -15.50000000000000000, 0.000000000000000000, -22.50000000000000000 ) ) ;
#5940=ADVANCED_FACE ( 'NONE', ( #9107 ), #13295, .T. ) ;
#5948=EDGE_CURVE ( 'NONE', #9306, #13359, #4614, .T. ) ;
#5962=CARTESIAN_POINT ( 'NONE',  ( 15.50000000000000000, -5.000000000000000000, -22.50000000000000000 ) ) ;
#5963=CARTESIAN_POINT ( 'NONE',  ( 14.25000000000000000, -2.500000000000000000, 23.22168783648699986 ) ) ;
#5970=CARTESIAN_POINT ( 'NONE',  ( -16.75000000000000000, -2.500000000000000000, 21.77831216351300014 ) ) ;
#5977=ORIENTED_EDGE ( 'NONE', *, *, #5383, .T. ) ;
#5990=B_SPLINE_CURVE_WITH_KNOTS ( 'NONE', 3,
 ( #6716, #10252, #12377, #4223, #6417, #2912 ),
 .UNSPECIFIED., .F., .F.,
 ( 4, 2, 4 ),
 ( 0.0002380763768115301549, 0.7291065797294569162, 1.457975083082102330 ),
 .UNSPECIFIED. ) ;
#5993=DIRECTION ( 'NONE',  ( -0.4999999999999832356, 0.000000000000000000, -0.8660254037844483666 ) ) ;
#6002=DIRECTION ( 'NONE',  ( 1.000000000000000000, -0.000000000000000000, 1.224646799147353207E-16 ) ) ;
#6005=DIRECTION ( 'NONE',  ( 0.000000000000000000, 0.000000000000000000, 1.000000000000000000 ) ) ;
#6014=CARTESIAN_POINT ( 'NONE',  ( 23.25000000000000000, -5.000000000000000000, 27.00000000000000000 ) ) ;
#6045=VECTOR ( 'NONE', #8166, 1000.000000000000000 ) ;
#6051=DIRECTION ( 'NONE',  ( 0.000000000000000000, 1.000000000000000000, 0.000000000000000000 ) ) ;
#6070=FILL_AREA_STYLE_COLOUR ( '', #14423 ) ;
#6083=VECTOR ( 'NONE', #589, 999.9999999999998863 ) ;
#6087=DIRECTION ( 'NONE',  ( 0.000000000000000000, 0.000000000000000000, 1.000000000000000000 ) ) ;
#6091=CARTESIAN_POINT ( 'NONE',  ( -16.75000000000000000, -0.2038245569916330158, 23.22168783648699986 ) ) ;
#6093=CARTESIAN_POINT ( 'NONE',  ( 15.50000000000000000, -0.4000000000005274892, -22.50000000000000000 ) ) ;
#6097=DIRECTION ( 'NONE',  ( 0.000000000000000000, -1.000000000000000000, -0.000000000000000000 ) ) ;
#6100=AXIS2_PLACEMENT_3D ( 'NONE', #1322, #1485, #164 ) ;
#6110=AXIS2_PLACEMENT_3D ( 'NONE', #3696, #9213, #13953 ) ;
#6111=PLANE ( 'NONE',  #14696 ) ;
#6113=ADVANCED_FACE ( 'NONE', ( #2356 ), #5876, .F. ) ;
#6133=COLOUR_RGB ( '', 0.09019608, 0.27058824, 0.51372549) ;
#6147=ADVANCED_FACE ( 'NONE', ( #10497, #9339, #14078, #13154, #11904 ), #9407, .F. ) ;
#6178=ORIENTED_EDGE ( 'NONE', *, *, #9061, .F. ) ;
#6187=FACE_OUTER_BOUND ( 'NONE', #5779, .T. ) ;
#6209=ORIENTED_EDGE ( 'NONE', *, *, #6528, .T. ) ;
#6214=ORIENTED_EDGE ( 'NONE', *, *, #7553, .F. ) ;
#6216=EDGE_CURVE ( 'NONE', #3055, #382, #14761, .T. ) ;
#6219=EDGE_CURVE ( 'NONE', #1114, #3042, #1663, .T. ) ;
#6225=EDGE_CURVE ( 'NONE', #7739, #13195, #11072, .T. ) ;
#6227=LINE ( 'NONE', #10789, #11244 ) ;
#6228=ORIENTED_EDGE ( 'NONE', *, *, #6501, .F. ) ;
#6230=VERTEX_POINT ( 'NONE', #11124 ) ;
#6235=ADVANCED_FACE ( 'NONE', ( #5228 ), #1633, .T. ) ;
#6277=CARTESIAN_POINT ( 'NONE',  ( -15.50000000000000000, -2.500000000000000000, 23.94337567297399971 ) ) ;
#6282=ORIENTED_EDGE ( 'NONE', *, *, #12466, .T. ) ;
#6283=EDGE_LOOP ( 'NONE', ( #12201, #5048, #14797, #3361, #5132, #8090 ) ) ;
#6287=CIRCLE ( 'NONE', #15157, 3.300000002979700753 ) ;
#6294=CARTESIAN_POINT ( 'NONE',  ( -14.25000000000000000, -2.500000000000000000, 21.77831216351300014 ) ) ;
#6298=CARTESIAN_POINT ( 'NONE',  ( -14.25000000000000000, -0.2038245569916330158, -21.77831216351300014 ) ) ;
#6300=CYLINDRICAL_SURFACE ( 'NONE', #7311, 3.499999999999999556 ) ;
#6302=CARTESIAN_POINT ( 'NONE',  ( -15.08757311576351690, -0.3152598339557960427, 23.70526090033903444 ) ) ;
#6320=EDGE_CURVE ( 'NONE', #12945, #9206, #5163, .T. ) ;
#6337=CARTESIAN_POINT ( 'NONE',  ( -15.50000000000000000, -1.037157890325000054, 19.00000000000000000 ) ) ;
#6364=ORIENTED_EDGE ( 'NONE', *, *, #12670, .T. ) ;
#6376=DIRECTION ( 'NONE',  ( 1.060575238724892987E-16, 0.5000000000000199840, -0.8660254037844271613 ) ) ;
#6378=FACE_BOUND ( 'NONE', #8683, .T. ) ;
#6384=EDGE_LOOP ( 'NONE', ( #13853, #14704, #4189, #7942 ) ) ;
#6389=AXIS2_PLACEMENT_3D ( 'NONE', #8549, #7174, #14437 ) ;
#6396=CARTESIAN_POINT ( 'NONE',  ( 15.50000000000000000, -0.1999999999999999556, -22.50000000000000000 ) ) ;
#6399=DIRECTION ( 'NONE',  ( 0.000000000000000000, 0.000000000000000000, 1.000000000000000000 ) ) ;
#6401=CARTESIAN_POINT ( 'NONE',  ( 23.25000000000000000, 0.000000000000000000, 27.00000000000000000 ) ) ;
#6417=CARTESIAN_POINT ( 'NONE',  ( 15.29633693294940500, -0.2717122460100945269, 23.82579074638835692 ) ) ;
#6431=FACE_OUTER_BOUND ( 'NONE', #14196, .T. ) ;
#6444=EDGE_CURVE ( 'NONE', #6610, #4486, #6858, .T. ) ;
#6450=VERTEX_POINT ( 'NONE', #5466 ) ;
#6456=ORIENTED_EDGE ( 'NONE', *, *, #9705, .F. ) ;
#6460=FACE_BOUND ( 'NONE', #7446, .T. ) ;
#6466=CARTESIAN_POINT ( 'NONE',  ( 16.75000000000000000, -0.2038245569916320166, 21.77831216351300014 ) ) ;
#6467=CARTESIAN_POINT ( 'NONE',  ( -15.50000000000000000, -0.1999999999999999556, 21.05000000000000071 ) ) ;
#6472=ORIENTED_EDGE ( 'NONE', *, *, #214, .T. ) ;
#6477=FACE_OUTER_BOUND ( 'NONE', #9592, .T. ) ;
#6486=ADVANCED_FACE ( 'NONE', ( #6709 ), #3500, .F. ) ;
#6494=CARTESIAN_POINT ( 'NONE',  ( -15.50000000000000000, 0.000000000000000000, -18.50000000000000000 ) ) ;
#6501=EDGE_CURVE ( 'NONE', #14030, #10998, #7091, .T. ) ;
#6503=ORIENTED_EDGE ( 'NONE', *, *, #11722, .F. ) ;
#6508=EDGE_CURVE ( 'NONE', #5722, #5825, #7357, .T. ) ;
#6513=EDGE_CURVE ( 'NONE', #14415, #59, #13136, .T. ) ;
#6514=DIRECTION ( 'NONE',  ( 0.000000000000000000, 0.000000000000000000, 1.000000000000000000 ) ) ;
#6516=DIRECTION ( 'NONE',  ( -1.000000000000000000, 0.000000000000000000, 0.000000000000000000 ) ) ;
#6524=LINE ( 'NONE', #3094, #8758 ) ;
#6528=EDGE_CURVE ( 'NONE', #1408, #13195, #4914, .T. ) ;
#6545=CARTESIAN_POINT ( 'NONE',  ( -15.50000000000000000, -0.1999999999999999556, -21.05000000000000071 ) ) ;
#6551=EDGE_LOOP ( 'NONE', ( #7992, #7689, #9098, #14950, #14046, #5635 ) ) ;
#6554=CIRCLE ( 'NONE', #3069, 3.499999999999999556 ) ;
#6562=CARTESIAN_POINT ( 'NONE',  ( 16.75000000000000000, -2.500000000000000000, 21.77831216351300014 ) ) ;
#6573=AXIS2_PLACEMENT_3D ( 'NONE', #13193, #9839, #2553 ) ;
#6575=VECTOR ( 'NONE', #5776, 1000.000000000000000 ) ;
#6579=DIRECTION ( 'NONE',  ( -1.000000000000000000, 0.000000000000000000, 0.000000000000000000 ) ) ;
#6581=LINE ( 'NONE', #14924, #10552 ) ;
#6586=( GEOMETRIC_REPRESENTATION_CONTEXT ( 3 ) GLOBAL_UNCERTAINTY_ASSIGNED_CONTEXT ( ( #2025 ) ) GLOBAL_UNIT_ASSIGNED_CONTEXT ( ( #8770, #2797, #395 ) ) REPRESENTATION_CONTEXT ( 'NONE', 'WORKASPACE' ) );
#6589=ORIENTED_EDGE ( 'NONE', *, *, #9901, .T. ) ;
#6595=ADVANCED_FACE ( 'NONE', ( #10635 ), #2487, .T. ) ;
#6600=DIRECTION ( 'NONE',  ( -0.8660254037844482555, 0.000000000000000000, 0.4999999999999831801 ) ) ;
#6610=VERTEX_POINT ( 'NONE', #9393 ) ;
#6618=ADVANCED_FACE ( 'NONE', ( #9318 ), #14060, .F. ) ;
#6658=DIRECTION ( 'NONE',  ( 0.000000000000000000, 1.000000000000000000, 0.000000000000000000 ) ) ;
#6662=DIRECTION ( 'NONE',  ( 0.000000000000000000, 0.000000000000000000, -1.000000000000000000 ) ) ;
#6681=ORIENTED_EDGE ( 'NONE', *, *, #4515, .T. ) ;
#6688=CARTESIAN_POINT ( 'NONE',  ( -16.74999999999999289, -0.3152037684892574076, 22.74589050208021490 ) ) ;
#6695=CARTESIAN_POINT ( 'NONE',  ( 16.75000000000000000, -0.3156864504677172611, 22.74361999681791602 ) ) ;
#6700=ORIENTED_EDGE ( 'NONE', *, *, #13303, .F. ) ;
#6709=FACE_OUTER_BOUND ( 'NONE', #15293, .T. ) ;
#6710=EDGE_CURVE ( 'NONE', #3939, #3973, #7180, .T. ) ;
#6713=CYLINDRICAL_SURFACE ( 'NONE', #2838, 3.499999999999999556 ) ;
#6716=CARTESIAN_POINT ( 'NONE',  ( 14.25000000000000000, -0.2038245569916330158, 23.22168783648699986 ) ) ;
#6726=CARTESIAN_POINT ( 'NONE',  ( 15.50000000000000000, -0.4000000000000000222, 22.50000000000000000 ) ) ;
#6729=DIRECTION ( 'NONE',  ( 0.000000000000000000, 1.000000000000000000, 0.000000000000000000 ) ) ;
#6730=AXIS2_PLACEMENT_3D ( 'NONE', #6562, #14903, #647 ) ;
#6737=DIRECTION ( 'NONE',  ( 0.000000000000000000, 0.000000000000000000, 1.000000000000000000 ) ) ;
#6741=DIRECTION ( 'NONE',  ( 0.000000000000000000, 0.000000000000000000, 1.000000000000000000 ) ) ;
#6748=ORIENTED_EDGE ( 'NONE', *, *, #10523, .T. ) ;
#6765=DIRECTION ( 'NONE',  ( 0.000000000000000000, 0.000000000000000000, 1.000000000000000000 ) ) ;
#6767=CARTESIAN_POINT ( 'NONE',  ( -16.54686605390241994, -0.2715358723599897717, -21.66103272505201360 ) ) ;
#6773=ORIENTED_EDGE ( 'NONE', *, *, #5748, .F. ) ;
#6782=CARTESIAN_POINT ( 'NONE',  ( 15.50000000000000000, -1.037157890325000054, -22.50000000000000000 ) ) ;
#6799=DIRECTION ( 'NONE',  ( 0.000000000000000000, 0.5000000000000199840, 0.8660254037844271613 ) ) ;
#6803=VECTOR ( 'NONE', #5053, 1000.000000000000000 ) ;
#6809=LINE ( 'NONE', #9181, #49 ) ;
#6810=VERTEX_POINT ( 'NONE', #11257 ) ;
#6823=FACE_OUTER_BOUND ( 'NONE', #6384, .T. ) ;
#6825=AXIS2_PLACEMENT_3D ( 'NONE', #8998, #3252, #2092 ) ;
#6830=VERTEX_POINT ( 'NONE', #5448 ) ;
#6831=VERTEX_POINT ( 'NONE', #5523 ) ;
#6841=LINE ( 'NONE', #10313, #1120 ) ;
#6845=DIRECTION ( 'NONE',  ( 0.000000000000000000, 1.000000000000000000, 0.000000000000000000 ) ) ;
#6849=ORIENTED_EDGE ( 'NONE', *, *, #9061, .T. ) ;
#6858=LINE ( 'NONE', #11500, #4627 ) ;
#6864=LINE ( 'NONE', #3593, #8606 ) ;
#6877=AXIS2_PLACEMENT_3D ( 'NONE', #1694, #7606, #12329 ) ;
#6895=EDGE_CURVE ( 'NONE', #14169, #11388, #13593, .T. ) ;
#6897=( NAMED_UNIT ( * ) SI_UNIT ( $, .STERADIAN. ) SOLID_ANGLE_UNIT ( ) );
#6899=DIRECTION ( 'NONE',  ( -0.8660254037844485886, 0.000000000000000000, -0.4999999999999827360 ) ) ;
#6902=DIRECTION ( 'NONE',  ( 0.000000000000000000, 0.5000000000000189848, 0.8660254037844277164 ) ) ;
#6904=VERTEX_POINT ( 'NONE', #3645 ) ;
#6914=CARTESIAN_POINT ( 'NONE',  ( -15.50000000000000000, -2.500000000000000000, 21.05662432702600029 ) ) ;
#6919=CARTESIAN_POINT ( 'NONE',  ( -14.25000000000000000, -2.500000000000000000, 23.22168783648699986 ) ) ;
#6927=CARTESIAN_POINT ( 'NONE',  ( 15.50000000000000000, -0.2038245569916610489, 21.05662432702600029 ) ) ;
#6933=DIRECTION ( 'NONE',  ( 1.000000000000000000, 0.000000000000000000, 0.000000000000000000 ) ) ;
#6934=CARTESIAN_POINT ( 'NONE',  ( 16.75000000000000000, -2.500000000000000000, -21.77831216351300014 ) ) ;
#6946=CARTESIAN_POINT ( 'NONE',  ( -15.50000000000000000, -2.500000000000000000, -21.05662432702600029 ) ) ;
#6961=DIRECTION ( 'NONE',  ( 0.000000000000000000, 0.000000000000000000, 1.000000000000000000 ) ) ;
#6972=VERTEX_POINT ( 'NONE', #64 ) ;
#6980=CYLINDRICAL_SURFACE ( 'NONE', #3829, 4.000000000000000000 ) ;
#7003=CARTESIAN_POINT ( 'NONE',  ( 14.45366306705350112, -0.2717122460102528447, 21.66072723692567692 ) ) ;
#7012=ORIENTED_EDGE ( 'NONE', *, *, #9522, .T. ) ;
#7014=ORIENTED_EDGE ( 'NONE', *, *, #7216, .T. ) ;
#7016=DIRECTION ( 'NONE',  ( 0.000000000000000000, 0.000000000000000000, 1.000000000000000000 ) ) ;
#7020=CIRCLE ( 'NONE', #12696, 4.000000000000000888 ) ;
#7029=DIRECTION ( 'NONE',  ( -0.8660254037844482555, 0.000000000000000000, 0.4999999999999831801 ) ) ;
#7031=AXIS2_PLACEMENT_3D ( 'NONE', #5736, #5509, #8133 ) ;
#7033=PRODUCT_CONTEXT ( 'NONE', #2468, 'mechanical' ) ;
#7035=CIRCLE ( 'NONE', #335, 1.449999999999999956 ) ;
#7049=CARTESIAN_POINT ( 'NONE',  ( -23.24999999999999289, -5.000000000000000000, 27.00000000000000000 ) ) ;
#7052=DIRECTION ( 'NONE',  ( -0.000000000000000000, 1.000000000000000000, -0.000000000000000000 ) ) ;
#7065=ADVANCED_FACE ( 'NONE', ( #11864 ), #13791, .T. ) ;
#7068=CIRCLE ( 'NONE', #4324, 3.499999999999999556 ) ;
#7071=CARTESIAN_POINT ( 'NONE',  ( -16.75000000000000000, -2.500000000000000000, 23.22168783648699986 ) ) ;
#7074=CARTESIAN_POINT ( 'NONE',  ( 15.50000000000000000, 0.000000000000000000, -18.50000000000000000 ) ) ;
#7081=ORIENTED_EDGE ( 'NONE', *, *, #12184, .F. ) ;
#7087=ADVANCED_FACE ( 'NONE', ( #7143 ), #11787, .F. ) ;
#7088=CARTESIAN_POINT ( 'NONE',  ( -16.33565937784311828, -0.3156604612129161880, -23.46090750622545684 ) ) ;
#7090=CARTESIAN_POINT ( 'NONE',  ( -14.25000000000000000, -0.3156864504677174277, 22.74361999681791247 ) ) ;
#7091=LINE ( 'NONE', #10715, #15001 ) ;
#7107=AXIS2_PLACEMENT_3D ( 'NONE', #12981, #14206, #2257 ) ;
#7126=CARTESIAN_POINT ( 'NONE',  ( 15.50000000000000000, -5.000000000000000000, -22.50000000000000000 ) ) ;
#7133=CARTESIAN_POINT ( 'NONE',  ( -14.25000000000000000, -0.2038245569916330158, -23.22168783648699986 ) ) ;
#7143=FACE_OUTER_BOUND ( 'NONE', #1610, .T. ) ;
#7156=ORIENTED_EDGE ( 'NONE', *, *, #4313, .F. ) ;
#7164=CARTESIAN_POINT ( 'NONE',  ( -14.24999999999999822, -0.3152037684892594616, 22.25410949791978510 ) ) ;
#7174=DIRECTION ( 'NONE',  ( 0.000000000000000000, 1.000000000000000000, 0.000000000000000000 ) ) ;
#7178=EDGE_LOOP ( 'NONE', ( #5171, #7598, #8288, #12017 ) ) ;
#7179=CARTESIAN_POINT ( 'NONE',  ( 16.75000000000000000, -2.500000000000000000, 21.77831216351300014 ) ) ;
#7180=B_SPLINE_CURVE_WITH_KNOTS ( 'NONE', 3,
 ( #2800, #7552, #1559, #12351, #1713, #13208 ),
 .UNSPECIFIED., .F., .F.,
 ( 4, 2, 4 ),
 ( 0.0002380763768132232450, 0.7291065797294586925, 1.457975083082104106 ),
 .UNSPECIFIED. ) ;
#7185=CARTESIAN_POINT ( 'NONE',  ( 15.50000000000000000, -0.2000000000000000111, 22.50000000000000000 ) ) ;
#7197=EDGE_LOOP ( 'NONE', ( #12237, #1279, #14837, #5403 ) ) ;
#7201=FACE_OUTER_BOUND ( 'NONE', #14418, .T. ) ;
#7216=EDGE_CURVE ( 'NONE', #1184, #5656, #11331, .T. ) ;
#7219=LINE ( 'NONE', #219, #14807 ) ;
#7228=VERTEX_POINT ( 'NONE', #6294 ) ;
#7232=FACE_OUTER_BOUND ( 'NONE', #3322, .T. ) ;
#7236=CARTESIAN_POINT ( 'NONE',  ( 15.50000000000000000, -1.037157890325000054, -19.00000000000000000 ) ) ;
#7239=CARTESIAN_POINT ( 'NONE',  ( 15.50000000000000000, -2.500000000000000000, 21.05662432702600029 ) ) ;
#7240=CARTESIAN_POINT ( 'NONE',  ( -15.08757311576351334, -0.3152598339557977081, -21.29473909966096556 ) ) ;
#7242=ORIENTED_EDGE ( 'NONE', *, *, #1173, .T. ) ;
#7246=VERTEX_POINT ( 'NONE', #13414 ) ;
#7250=ORIENTED_EDGE ( 'NONE', *, *, #3843, .T. ) ;
#7254=DIRECTION ( 'NONE',  ( 0.000000000000000000, 0.000000000000000000, 1.000000000000000000 ) ) ;
#7256=ADVANCED_FACE ( 'NONE', ( #13493 ), #2857, .F. ) ;
#7257=DIRECTION ( 'NONE',  ( 0.000000000000000000, 0.000000000000000000, 1.000000000000000000 ) ) ;
#7261=ORIENTED_EDGE ( 'NONE', *, *, #6513, .T. ) ;
#7268=ORIENTED_EDGE ( 'NONE', *, *, #1916, .F. ) ;
#7279=DIRECTION ( 'NONE',  ( 0.000000000000000000, 0.000000000000000000, 1.000000000000000000 ) ) ;
#7284=CARTESIAN_POINT ( 'NONE',  ( -16.75000000000000000, -2.500000000000000000, -21.77831216351300014 ) ) ;
#7311=AXIS2_PLACEMENT_3D ( 'NONE', #4901, #9606, #3719 ) ;
#7319=LINE ( 'NONE', #11963, #7578 ) ;
#7322=VERTEX_POINT ( 'NONE', #825 ) ;
#7327=ORIENTED_EDGE ( 'NONE', *, *, #13303, .T. ) ;
#7340=ORIENTED_EDGE ( 'NONE', *, *, #7747, .T. ) ;
#7344=CIRCLE ( 'NONE', #3613, 4.000000000000001776 ) ;
#7353=CARTESIAN_POINT ( 'NONE',  ( -15.50000000000000000, -0.2000000000000000111, -19.20000000000052509 ) ) ;
#7357=CIRCLE ( 'NONE', #7839, 4.000000000000000000 ) ;
#7365=CARTESIAN_POINT ( 'NONE',  ( -15.50000000000000000, -1.037157890325000054, -26.50000000000000000 ) ) ;
#7372=VECTOR ( 'NONE', #7029, 1000.000000000000114 ) ;
#7374=ORIENTED_EDGE ( 'NONE', *, *, #9789, .T. ) ;
#7377=ADVANCED_FACE ( 'NONE', ( #7201 ), #3462, .T. ) ;
#7381=CARTESIAN_POINT ( 'NONE',  ( 14.45313394609757296, -0.2715358723599907709, -21.66103272505201005 ) ) ;
#7386=EDGE_LOOP ( 'NONE', ( #11359, #4652 ) ) ;
#7389=VERTEX_POINT ( 'NONE', #8194 ) ;
#7391=ORIENTED_EDGE ( 'NONE', *, *, #3174, .F. ) ;
#7392=LINE ( 'NONE', #12116, #5576 ) ;
#7395=CYLINDRICAL_SURFACE ( 'NONE', #15226, 3.499999999999999556 ) ;
#7405=DIRECTION ( 'NONE',  ( 0.000000000000000000, 0.000000000000000000, 1.000000000000000000 ) ) ;
#7433=CARTESIAN_POINT ( 'NONE',  ( 14.25000000000000000, -0.2038245569916330158, -21.77831216351300014 ) ) ;
#7436=DIRECTION ( 'NONE',  ( 0.000000000000000000, -0.000000000000000000, 1.000000000000000000 ) ) ;
#7446=EDGE_LOOP ( 'NONE', ( #2384, #14748 ) ) ;
#7448=EDGE_CURVE ( 'NONE', #13359, #9306, #8609, .T. ) ;
#7460=ORIENTED_EDGE ( 'NONE', *, *, #13577, .T. ) ;
#7463=CARTESIAN_POINT ( 'NONE',  ( 15.50000000000000000, -0.4000000000000000222, 22.50000000000000000 ) ) ;
#7465=EDGE_CURVE ( 'NONE', #1114, #9632, #674, .T. ) ;
#7480=CARTESIAN_POINT ( 'NONE',  ( 15.50000000000000000, -5.000000000000000000, 22.50000000000000000 ) ) ;
#7484=ORIENTED_EDGE ( 'NONE', *, *, #2052, .T. ) ;
#7508=MECHANICAL_DESIGN_GEOMETRIC_PRESENTATION_REPRESENTATION('',(#796),#14919);
#7520=VERTEX_POINT ( 'NONE', #10028 ) ;
#7531=FACE_OUTER_BOUND ( 'NONE', #12236, .T. ) ;
#7532=SURFACE_SIDE_STYLE ('',( #13269 ) ) ;
#7533=CARTESIAN_POINT ( 'NONE',  ( -23.25000000000000000, 0.000000000000000000, -27.00000000000000000 ) ) ;
#7536=CARTESIAN_POINT ( 'NONE',  ( -14.45366306705349757, -0.2717122460102549542, 23.33927276307431242 ) ) ;
#7543=ORIENTED_EDGE ( 'NONE', *, *, #3562, .F. ) ;
#7547=DIRECTION ( 'NONE',  ( 0.000000000000000000, 0.000000000000000000, 1.000000000000000000 ) ) ;
#7552=CARTESIAN_POINT ( 'NONE',  ( 16.54686605390242349, -0.2715358723599871626, 21.66103272505201716 ) ) ;
#7553=EDGE_CURVE ( 'NONE', #7322, #6830, #2906, .T. ) ;
#7560=ADVANCED_FACE ( 'NONE', ( #5165, #9946 ), #2824, .T. ) ;
#7572=DIRECTION ( 'NONE',  ( 0.000000000000000000, 1.000000000000000000, 0.000000000000000000 ) ) ;
#7578=VECTOR ( 'NONE', #12048, 1000.000000000000000 ) ;
#7585=DIRECTION ( 'NONE',  ( 0.000000000000000000, 0.000000000000000000, 1.000000000000000000 ) ) ;
#7595=AXIS2_PLACEMENT_3D ( 'NONE', #2054, #11520, #4306 ) ;
#7598=ORIENTED_EDGE ( 'NONE', *, *, #5464, .F. ) ;
#7603=CARTESIAN_POINT ( 'NONE',  ( 23.25000000000000000, 0.000000000000000000, 27.00000000000000000 ) ) ;
#7606=DIRECTION ( 'NONE',  ( -0.4999999999999832356, 0.000000000000000000, 0.8660254037844483666 ) ) ;
#7610=DIRECTION ( 'NONE',  ( 0.000000000000000000, 1.000000000000000000, 0.000000000000000000 ) ) ;
#7618=ORIENTED_EDGE ( 'NONE', *, *, #6513, .F. ) ;
#7622=DIRECTION ( 'NONE',  ( 0.000000000000000000, 1.000000000000000000, 0.000000000000000000 ) ) ;
#7634=DIRECTION ( 'NONE',  ( 0.000000000000000000, 1.000000000000000000, 0.000000000000000000 ) ) ;
#7641=EDGE_LOOP ( 'NONE', ( #5410, #1318, #11491, #11755, #5534, #14671 ) ) ;
#7655=ORIENTED_EDGE ( 'NONE', *, *, #490, .T. ) ;
#7666=CARTESIAN_POINT ( 'NONE',  ( 15.50000000000000000, -2.500000000000000000, -23.94337567297399971 ) ) ;
#7682=FACE_OUTER_BOUND ( 'NONE', #10408, .T. ) ;
#7686=DIRECTION ( 'NONE',  ( 0.000000000000000000, 1.000000000000000000, 0.000000000000000000 ) ) ;
#7689=ORIENTED_EDGE ( 'NONE', *, *, #14731, .T. ) ;
#7704=ORIENTED_EDGE ( 'NONE', *, *, #7448, .T. ) ;
#7719=ORIENTED_EDGE ( 'NONE', *, *, #5074, .T. ) ;
#7721=EDGE_CURVE ( 'NONE', #4925, #3944, #186, .T. ) ;
#7727=EDGE_CURVE ( 'NONE', #51, #10402, #11345, .T. ) ;
#7736=DIRECTION ( 'NONE',  ( 0.000000000000000000, 0.000000000000000000, -1.000000000000000000 ) ) ;
#7739=VERTEX_POINT ( 'NONE', #4370 ) ;
#7741=ADVANCED_FACE ( 'NONE', ( #3274 ), #10399, .F. ) ;
#7747=EDGE_CURVE ( 'NONE', #10998, #7389, #2110, .T. ) ;
#7755=FILL_AREA_STYLE ('',( #9910 ) ) ;
#7756=LINE ( 'NONE', #680, #634 ) ;
#7757=DIRECTION ( 'NONE',  ( -0.8660254037844485886, 0.000000000000000000, -0.4999999999999827360 ) ) ;
#7760=CARTESIAN_POINT ( 'NONE',  ( -15.50000000000000000, -0.4000000000000000222, 22.50000000000000000 ) ) ;
#7762=ORIENTED_EDGE ( 'NONE', *, *, #4485, .T. ) ;
#7772=CARTESIAN_POINT ( 'NONE',  ( 15.50000000000000000, 0.000000000000000000, 26.50000000000000000 ) ) ;
#7777=CARTESIAN_POINT ( 'NONE',  ( 15.50000000000000000, -0.4000000000005274892, -19.20000000000052864 ) ) ;
#7778=VECTOR ( 'NONE', #2966, 1000.000000000000000 ) ;
#7809=ADVANCED_FACE ( 'NONE', ( #12894 ), #2259, .F. ) ;
#7823=AXIS2_PLACEMENT_3D ( 'NONE', #11049, #5001, #3837 ) ;
#7825=( LENGTH_UNIT ( ) NAMED_UNIT ( * ) SI_UNIT ( .MILLI., .METRE. ) );
#7827=CYLINDRICAL_SURFACE ( 'NONE', #10277, 4.000000000000000000 ) ;
#7829=DIRECTION ( 'NONE',  ( 0.4999999999999827360, 0.000000000000000000, -0.8660254037844485886 ) ) ;
#7830=EDGE_CURVE ( 'NONE', #3116, #7520, #14890, .T. ) ;
#7839=AXIS2_PLACEMENT_3D ( 'NONE', #5935, #4833, #11648 ) ;
#7840=FACE_OUTER_BOUND ( 'NONE', #5508, .T. ) ;
#7853=DIRECTION ( 'NONE',  ( 0.000000000000000000, 1.000000000000000000, 0.000000000000000000 ) ) ;
#7854=ORIENTED_EDGE ( 'NONE', *, *, #2143, .T. ) ;
#7859=CARTESIAN_POINT ( 'NONE',  ( 16.75000000000000000, -2.500000000000000000, 23.22168783648699986 ) ) ;
#7864=DIRECTION ( 'NONE',  ( 0.000000000000000000, 1.000000000000000000, 0.000000000000000000 ) ) ;
#7866=DIRECTION ( 'NONE',  ( 0.000000000000000000, 0.000000000000000000, 1.000000000000000000 ) ) ;
#7881=AXIS2_PLACEMENT_3D ( 'NONE', #4445, #13903, #2488 ) ;
#7884=CARTESIAN_POINT ( 'NONE',  ( -15.50000000000000000, 0.000000000000000000, 26.50000000000000000 ) ) ;
#7894=CARTESIAN_POINT ( 'NONE',  ( -14.25000000000000000, -0.2038245569916330158, 21.77831216351300014 ) ) ;
#7897=CARTESIAN_POINT ( 'NONE',  ( -15.50000000000000000, -0.2000000000000000111, -22.50000000000000000 ) ) ;
#7900=CARTESIAN_POINT ( 'NONE',  ( -16.75000000000000000, -2.500000000000000000, -23.22168783648699986 ) ) ;
#7903=ORIENTED_EDGE ( 'NONE', *, *, #2505, .F. ) ;
#7909=FACE_BOUND ( 'NONE', #14396, .T. ) ;
#7911=CARTESIAN_POINT ( 'NONE',  ( 15.50000000000000000, -1.037157890325000054, 18.50000000000000000 ) ) ;
#7913=DIRECTION ( 'NONE',  ( 0.000000000000000000, 0.000000000000000000, 1.000000000000000000 ) ) ;
#7916=CARTESIAN_POINT ( 'NONE',  ( 15.91242688423647600, -0.3152598339557935447, -21.29473909966096556 ) ) ;
#7933=DIRECTION ( 'NONE',  ( 0.000000000000000000, 0.000000000000000000, 1.000000000000000000 ) ) ;
#7942=ORIENTED_EDGE ( 'NONE', *, *, #10258, .T. ) ;
#7944=DIRECTION ( 'NONE',  ( 0.000000000000000000, 0.000000000000000000, -1.000000000000000000 ) ) ;
#7948=LINE ( 'NONE', #11297, #12554 ) ;
#7953=SURFACE_SIDE_STYLE ('',( #14008 ) ) ;
#7971=ORIENTED_EDGE ( 'NONE', *, *, #9705, .T. ) ;
#7973=ORIENTED_EDGE ( 'NONE', *, *, #345, .F. ) ;
#7975=ORIENTED_EDGE ( 'NONE', *, *, #4313, .T. ) ;
#7977=CONICAL_SURFACE ( 'NONE', #5024, 1732.050807568789651, 1.047197551196575871 ) ;
#7981=DIRECTION ( 'NONE',  ( 0.000000000000000000, 1.000000000000000000, 0.000000000000000000 ) ) ;
#7988=LINE ( 'NONE', #553, #4794 ) ;
#7991=AXIS2_PLACEMENT_3D ( 'NONE', #5914, #8216, #4572 ) ;
#7992=ORIENTED_EDGE ( 'NONE', *, *, #13299, .T. ) ;
#8000=AXIS2_PLACEMENT_3D ( 'NONE', #10654, #4619, #9564 ) ;
#8011=EDGE_LOOP ( 'NONE', ( #11528, #8703, #11409, #12078, #14645, #2894 ) ) ;
#8013=ORIENTED_EDGE ( 'NONE', *, *, #11591, .F. ) ;
#8022=CARTESIAN_POINT ( 'NONE',  ( -15.50000000000000000, -0.4000000000005236034, -22.50000000000000000 ) ) ;
#8024=DIRECTION ( 'NONE',  ( 0.000000000000000000, 1.000000000000000000, 0.000000000000000000 ) ) ;
#8028=CARTESIAN_POINT ( 'NONE',  ( 14.25000000000000000, -2.500000000000000000, -23.22168783648699986 ) ) ;
#8036=CIRCLE ( 'NONE', #6573, 4.000000000000000000 ) ;
#8046=ORIENTED_EDGE ( 'NONE', *, *, #5346, .T. ) ;
#8053=ORIENTED_EDGE ( 'NONE', *, *, #2625, .F. ) ;
#8059=VECTOR ( 'NONE', #15247, 1000.000000000000000 ) ;
#8067=CARTESIAN_POINT ( 'NONE',  ( 16.33565937784172917, -0.3156604612126716614, -21.53909249377372959 ) ) ;
#8079=SURFACE_SIDE_STYLE ('',( #3346 ) ) ;
#8080=CIRCLE ( 'NONE', #12059, 3.299999999999473577 ) ;
#8081=LINE ( 'NONE', #12819, #5511 ) ;
#8083=DIRECTION ( 'NONE',  ( 0.000000000000000000, 1.000000000000000000, 0.000000000000000000 ) ) ;
#8085=CARTESIAN_POINT ( 'NONE',  ( -15.50000000000000000, 0.000000000000000000, 22.50000000000000000 ) ) ;
#8086=DIRECTION ( 'NONE',  ( 0.000000000000000000, 1.000000000000000000, 0.000000000000000000 ) ) ;
#8090=ORIENTED_EDGE ( 'NONE', *, *, #14370, .T. ) ;
#8110=VERTEX_POINT ( 'NONE', #13442 ) ;
#8116=CARTESIAN_POINT ( 'NONE',  ( -15.08565937784311473, -0.3156604612129270127, 21.29584399676446083 ) ) ;
#8118=ORIENTED_EDGE ( 'NONE', *, *, #9815, .T. ) ;
#8130=CARTESIAN_POINT ( 'NONE',  ( 0.000000000000000000, -2.500000000000000000, 45.00000000000000000 ) ) ;
#8133=DIRECTION ( 'NONE',  ( -0.8660254037844485886, 0.000000000000000000, -0.4999999999999827360 ) ) ;
#8137=VERTEX_POINT ( 'NONE', #2239 ) ;
#8139=ORIENTED_EDGE ( 'NONE', *, *, #4658, .T. ) ;
#8144=DIRECTION ( 'NONE',  ( -0.8660254037844482555, 0.000000000000000000, 0.4999999999999831801 ) ) ;
#8151=CARTESIAN_POINT ( 'NONE',  ( -15.50000000000000000, -0.1999999999999999556, 22.50000000000000000 ) ) ;
#8155=AXIS2_PLACEMENT_3D ( 'NONE', #13850, #1825, #5568 ) ;
#8163=DIRECTION ( 'NONE',  ( 0.000000000000000000, 1.000000000000000000, 0.000000000000000000 ) ) ;
#8166=DIRECTION ( 'NONE',  ( 0.000000000000000000, 1.000000000000000000, 0.000000000000000000 ) ) ;
#8189=EDGE_LOOP ( 'NONE', ( #13319, #986, #4359, #11639, #4765, #7704 ) ) ;
#8194=CARTESIAN_POINT ( 'NONE',  ( 16.75000000000000000, -0.2038245569916320166, -21.77831216351300014 ) ) ;
#8205=EDGE_CURVE ( 'NONE', #8552, #4318, #12601, .T. ) ;
#8214=AXIS2_PLACEMENT_3D ( 'NONE', #11972, #3438, #7016 ) ;
#8216=DIRECTION ( 'NONE',  ( -0.4999999999999832356, 0.000000000000000000, 0.8660254037844483666 ) ) ;
#8230=ORIENTED_EDGE ( 'NONE', *, *, #7448, .F. ) ;
#8246=ORIENTED_EDGE ( 'NONE', *, *, #14917, .F. ) ;
#8272=CIRCLE ( 'NONE', #1324, 3.499999999999999556 ) ;
#8275=CARTESIAN_POINT ( 'NONE',  ( 15.50000000000000000, -0.1999999999999999556, 22.50000000000000000 ) ) ;
#8286=CARTESIAN_POINT ( 'NONE',  ( -15.50000000000000000, -5.000000000000000000, 26.50000000000000000 ) ) ;
#8288=ORIENTED_EDGE ( 'NONE', *, *, #13857, .T. ) ;
#8297=EDGE_CURVE ( 'NONE', #1915, #4436, #4812, .T. ) ;
#8328=ORIENTED_EDGE ( 'NONE', *, *, #8297, .T. ) ;
#8334=ORIENTED_EDGE ( 'NONE', *, *, #1335, .T. ) ;
#8340=VECTOR ( 'NONE', #5700, 1000.000000000000000 ) ;
#8375=B_SPLINE_CURVE_WITH_KNOTS ( 'NONE', 3,
 ( #9925, #8849, #13659, #6688, #12505, #14737 ),
 .UNSPECIFIED., .F., .F.,
 ( 4, 2, 4 ),
 ( 1.820537833122031213, 2.555393473688635453, 3.290249114255239693 ),
 .UNSPECIFIED. ) ;
#8376=CARTESIAN_POINT ( 'NONE',  ( -15.50000000000000000, -0.4000000000005236034, 22.50000000000000000 ) ) ;
#8381=DIRECTION ( 'NONE',  ( -1.000000000000000000, 0.000000000000000000, 0.000000000000000000 ) ) ;
#8389=ORIENTED_EDGE ( 'NONE', *, *, #10263, .F. ) ;
#8391=CARTESIAN_POINT ( 'NONE',  ( -15.50000000000000000, -0.2038245569916614930, -23.94337567297399971 ) ) ;
#8399=CARTESIAN_POINT ( 'NONE',  ( -15.50000000000000000, -5.000000000000000000, -22.50000000000000000 ) ) ;
#8407=CARTESIAN_POINT ( 'NONE',  ( -16.75000000000000000, -0.2038245569916330158, -21.77831216351300014 ) ) ;
#8409=EDGE_CURVE ( 'NONE', #4688, #6450, #7219, .T. ) ;
#8415=CARTESIAN_POINT ( 'NONE',  ( 14.25000000000000000, -0.2038245569916330158, 21.77831216351300014 ) ) ;
#8417=FACE_OUTER_BOUND ( 'NONE', #2082, .T. ) ;
#8432=EDGE_LOOP ( 'NONE', ( #7327, #2787, #2311, #11057 ) ) ;
#8438=CARTESIAN_POINT ( 'NONE',  ( -15.50000000000000000, -1.037157890325000054, 22.50000000000000000 ) ) ;
#8444=PRESENTATION_STYLE_ASSIGNMENT (( #4813 ) ) ;
#8471=AXIS2_PLACEMENT_3D ( 'NONE', #8130, #908, #2072 ) ;
#8473=ORIENTED_EDGE ( 'NONE', *, *, #3562, .T. ) ;
#8478=EDGE_CURVE ( 'NONE', #4688, #1915, #1697, .T. ) ;
#8484=ADVANCED_FACE ( 'NONE', ( #7531 ), #2940, .F. ) ;
#8518=CIRCLE ( 'NONE', #3554, 4.000000000000000000 ) ;
#8519=ORIENTED_EDGE ( 'NONE', *, *, #2177, .T. ) ;
#8529=ORIENTED_EDGE ( 'NONE', *, *, #7721, .T. ) ;
#8547=DIRECTION ( 'NONE',  ( 0.000000000000000000, 1.000000000000000000, 0.000000000000000000 ) ) ;
#8549=CARTESIAN_POINT ( 'NONE',  ( 15.50000000000000000, 0.000000000000000000, 22.50000000000000000 ) ) ;
#8552=VERTEX_POINT ( 'NONE', #4474 ) ;
#8561=CARTESIAN_POINT ( 'NONE',  ( -16.54633693294650953, -0.2717122460102549542, 21.66072723692568402 ) ) ;
#8562=CARTESIAN_POINT ( 'NONE',  ( 14.45366306705349402, -0.2717122460102546766, -23.33927276307431598 ) ) ;
#8566=CARTESIAN_POINT ( 'NONE',  ( 23.25000000000000000, 0.000000000000000000, -27.00000000000000000 ) ) ;
#8572=VECTOR ( 'NONE', #7572, 1000.000000000000000 ) ;
#8582=B_SPLINE_CURVE_WITH_KNOTS ( 'NONE', 3,
 ( #4273, #6767, #14883, #703, #13822, #627 ),
 .UNSPECIFIED., .F., .F.,
 ( 4, 2, 4 ),
 ( 0.0002380763768131538560, 0.7291065797294589146, 1.457975083082104550 ),
 .UNSPECIFIED. ) ;
#8585=AXIS2_PLACEMENT_3D ( 'NONE', #3350, #8083, #5853 ) ;
#8589=LINE ( 'NONE', #8656, #1392 ) ;
#8591=ORIENTED_EDGE ( 'NONE', *, *, #4774, .T. ) ;
#8598=AXIS2_PLACEMENT_3D ( 'NONE', #12617, #1979, #9038 ) ;
#8606=VECTOR ( 'NONE', #9326, 1000.000000000000114 ) ;
#8609=CIRCLE ( 'NONE', #429, 1.449999999999996403 ) ;
#8623=CARTESIAN_POINT ( 'NONE',  ( -15.50000000000000000, -2.500000000000000000, 23.94337567297399971 ) ) ;
#8624=FACE_OUTER_BOUND ( 'NONE', #1443, .T. ) ;
#8625=ORIENTED_EDGE ( 'NONE', *, *, #11200, .T. ) ;
#8626=CARTESIAN_POINT ( 'NONE',  ( -15.50000000000000000, -0.1999999999999999556, -23.94999999999999929 ) ) ;
#8636=CARTESIAN_POINT ( 'NONE',  ( -15.50000000000000000, -5.000000000000000000, 22.50000000000000000 ) ) ;
#8656=CARTESIAN_POINT ( 'NONE',  ( -15.50000000000000000, -2.500000000000000000, -23.94337567297399971 ) ) ;
#8659=DIRECTION ( 'NONE',  ( -1.000000000000000000, 0.000000000000000000, -0.000000000000000000 ) ) ;
#8675=CARTESIAN_POINT ( 'NONE',  ( 14.25000000000000000, -0.2038245569916330158, -21.77831216351300014 ) ) ;
#8683=EDGE_LOOP ( 'NONE', ( #11827, #5674 ) ) ;
#8703=ORIENTED_EDGE ( 'NONE', *, *, #12740, .T. ) ;
#8708=CIRCLE ( 'NONE', #12921, 4.000000000000000000 ) ;
#8710=CARTESIAN_POINT ( 'NONE',  ( 15.08757311576526128, -0.3152598339554911200, -23.70526090034004341 ) ) ;
#8711=B_SPLINE_CURVE_WITH_KNOTS ( 'NONE', 3,
 ( #8982, #8756, #14722, #3955, #13423, #12337 ),
 .UNSPECIFIED., .F., .F.,
 ( 4, 2, 4 ),
 ( 0.0002380763768114607659, 0.7291065797294573603, 1.457975083082103218 ),
 .UNSPECIFIED. ) ;
#8715=AXIS2_PLACEMENT_3D ( 'NONE', #4316, #6729, #5492 ) ;
#8728=AXIS2_PLACEMENT_3D ( 'NONE', #5431, #10598, #12862 ) ;
#8746=VECTOR ( 'NONE', #3192, 1000.000000000000000 ) ;
#8756=CARTESIAN_POINT ( 'NONE',  ( 16.54686605390242349, -0.2715358723599884394, -23.33896727494797929 ) ) ;
#8758=VECTOR ( 'NONE', #11242, 1000.000000000000114 ) ;
#8770=( LENGTH_UNIT ( ) NAMED_UNIT ( * ) SI_UNIT ( .MILLI., .METRE. ) );
#8789=EDGE_CURVE ( 'NONE', #1628, #15023, #14242, .T. ) ;
#8794=FACE_OUTER_BOUND ( 'NONE', #5027, .T. ) ;
#8805=STYLED_ITEM ( 'NONE', ( #11676 ), #330 ) ;
#8833=EDGE_CURVE ( 'NONE', #541, #7520, #13330, .T. ) ;
#8834=LINE ( 'NONE', #14720, #14718 ) ;
#8837=TOROIDAL_SURFACE ( 'NONE', #2389, 3.299999999999470024, 0.2000000000005275058 ) ;
#8849=CARTESIAN_POINT ( 'NONE',  ( -16.75000000000000355, -0.2715193793361416197, 22.01281590054916748 ) ) ;
#8855=LINE ( 'NONE', #11715, #154 ) ;
#8862=ORIENTED_EDGE ( 'NONE', *, *, #9522, .F. ) ;
#8871=CARTESIAN_POINT ( 'NONE',  ( 15.50000000000000000, -0.2038245569916610489, -23.94337567297399971 ) ) ;
#8872=DIRECTION ( 'NONE',  ( 0.000000000000000000, 1.000000000000000000, 0.000000000000000000 ) ) ;
#8881=EDGE_LOOP ( 'NONE', ( #3083, #12590, #3283, #10404 ) ) ;
#8886=VECTOR ( 'NONE', #12248, 1000.000000000000000 ) ;
#8892=LINE ( 'NONE', #12463, #10050 ) ;
#8901=PLANE ( 'NONE',  #1267 ) ;
#8909=DIRECTION ( 'NONE',  ( 0.000000000000000000, -0.000000000000000000, 1.000000000000000000 ) ) ;
#8913=ORIENTED_EDGE ( 'NONE', *, *, #3651, .T. ) ;
#8921=CARTESIAN_POINT ( 'NONE',  ( 15.50000000000000000, -1.037157890325000054, -22.50000000000000000 ) ) ;
#8944=FACE_OUTER_BOUND ( 'NONE', #10847, .T. ) ;
#8945=ORIENTED_EDGE ( 'NONE', *, *, #2913, .T. ) ;
#8950=ORIENTED_EDGE ( 'NONE', *, *, #6219, .T. ) ;
#8954=ADVANCED_FACE ( 'NONE', ( #6431 ), #2608, .T. ) ;
#8960=DIRECTION ( 'NONE',  ( 0.000000000000000000, 0.000000000000000000, 1.000000000000000000 ) ) ;
#8964=DIRECTION ( 'NONE',  ( 0.000000000000000000, 0.5000000000000189848, 0.8660254037844277164 ) ) ;
#8967=ADVANCED_FACE ( 'NONE', ( #12152 ), #1522, .F. ) ;
#8976=AXIS2_PLACEMENT_3D ( 'NONE', #13852, #15311, #12768 ) ;
#8982=CARTESIAN_POINT ( 'NONE',  ( 16.75000000000000000, -0.2038245569916320166, -23.22168783648699986 ) ) ;
#8989=ORIENTED_EDGE ( 'NONE', *, *, #15004, .F. ) ;
#8998=CARTESIAN_POINT ( 'NONE',  ( -15.50000000000000000, -1.037157890325000054, -22.50000000000000000 ) ) ;
#9003=ORIENTED_EDGE ( 'NONE', *, *, #11240, .T. ) ;
#9010=CARTESIAN_POINT ( 'NONE',  ( 15.50000000000000000, -0.2038245569916604938, 23.94337567297399971 ) ) ;
#9024=EDGE_CURVE ( 'NONE', #14169, #12927, #14779, .T. ) ;
#9031=DIRECTION ( 'NONE',  ( 0.000000000000000000, 0.000000000000000000, 1.000000000000000000 ) ) ;
#9034=DIRECTION ( 'NONE',  ( 0.000000000000000000, 0.000000000000000000, 1.000000000000000000 ) ) ;
#9038=DIRECTION ( 'NONE',  ( 0.000000000000000000, 0.000000000000000000, 1.000000000000000000 ) ) ;
#9052=AXIS2_PLACEMENT_3D ( 'NONE', #11596, #13996, #733 ) ;
#9056=EDGE_CURVE ( 'NONE', #5926, #6810, #216, .T. ) ;
#9061=EDGE_CURVE ( 'NONE', #1528, #7246, #1467, .T. ) ;
#9066=VECTOR ( 'NONE', #13403, 1000.000000000000114 ) ;
#9067=ORIENTED_EDGE ( 'NONE', *, *, #13046, .F. ) ;
#9072=FACE_OUTER_BOUND ( 'NONE', #14065, .T. ) ;
#9074=LINE ( 'NONE', #8921, #2544 ) ;
#9087=CIRCLE ( 'NONE', #10076, 3.499999999999999556 ) ;
#9098=ORIENTED_EDGE ( 'NONE', *, *, #2600, .T. ) ;
#9107=FACE_OUTER_BOUND ( 'NONE', #1316, .T. ) ;
#9118=ORIENTED_EDGE ( 'NONE', *, *, #13892, .T. ) ;
#9127=PLANE ( 'NONE',  #2116 ) ;
#9130=CARTESIAN_POINT ( 'NONE',  ( -15.50000000000000000, 0.000000000000000000, 22.50000000000000000 ) ) ;
#9152=B_SPLINE_CURVE_WITH_KNOTS ( 'NONE', 3,
 ( #8675, #7381, #5041, #9754, #14490, #13419 ),
 .UNSPECIFIED., .F., .F.,
 ( 4, 2, 4 ),
 ( 0.0002380763768132926339, 0.7291065797294586925, 1.457975083082104106 ),
 .UNSPECIFIED. ) ;
#9156=VERTEX_POINT ( 'NONE', #2440 ) ;
#9176=DIRECTION ( 'NONE',  ( 0.8660254037844485886, 0.000000000000000000, -0.4999999999999827360 ) ) ;
#9181=CARTESIAN_POINT ( 'NONE',  ( 15.50000000000000000, -2.500000000000000000, 21.05662432702600029 ) ) ;
#9186=FILL_AREA_STYLE_COLOUR ( '', #11035 ) ;
#9206=VERTEX_POINT ( 'NONE', #8415 ) ;
#9213=DIRECTION ( 'NONE',  ( 0.000000000000000000, 1.000000000000000000, 0.000000000000000000 ) ) ;
#9224=LINE ( 'NONE', #12729, #8746 ) ;
#9225=AXIS2_PLACEMENT_3D ( 'NONE', #6914, #1073, #8144 ) ;
#9242=CARTESIAN_POINT ( 'NONE',  ( 15.50000000000000000, -1.037157890325000054, -22.50000000000000000 ) ) ;
#9259=PLANE ( 'NONE',  #11050 ) ;
#9270=ORIENTED_EDGE ( 'NONE', *, *, #14893, .T. ) ;
#9286=VERTEX_POINT ( 'NONE', #8566 ) ;
#9300=CARTESIAN_POINT ( 'NONE',  ( -15.50000000000000000, -0.2038245569916614930, 21.05662432702600029 ) ) ;
#9306=VERTEX_POINT ( 'NONE', #14531 ) ;
#9309=VECTOR ( 'NONE', #10897, 1000.000000000000000 ) ;
#9318=FACE_OUTER_BOUND ( 'NONE', #4153, .T. ) ;
#9320=DIRECTION ( 'NONE',  ( 0.9375000000000004441, 0.000000000000000000, 0.3479852726768752902 ) ) ;
#9326=DIRECTION ( 'NONE',  ( -0.8660254037844482555, 0.000000000000000000, 0.4999999999999831801 ) ) ;
#9328=EDGE_LOOP ( 'NONE', ( #10628, #4723, #6773, #2153 ) ) ;
#9339=FACE_BOUND ( 'NONE', #687, .T. ) ;
#9342=AXIS2_PLACEMENT_3D ( 'NONE', #10927, #1539, #6514 ) ;
#9349=CARTESIAN_POINT ( 'NONE',  ( -14.45313394609757651, -0.2715358723599896051, 21.66103272505202781 ) ) ;
#9378=CARTESIAN_POINT ( 'NONE',  ( -15.50000000000000000, -0.4000000000005236034, 25.79999999999947136 ) ) ;
#9381=CARTESIAN_POINT ( 'NONE',  ( -16.75000000000000000, -2.500000000000000000, -21.77831216351300014 ) ) ;
#9390=CARTESIAN_POINT ( 'NONE',  ( 15.50000000000000000, -0.4000000000005274892, 25.79999999999946780 ) ) ;
#9391=CARTESIAN_POINT ( 'NONE',  ( 16.75000000000000000, -2.500000000000000000, -23.22168783648699986 ) ) ;
#9393=CARTESIAN_POINT ( 'NONE',  ( -14.25000000000000000, -2.500000000000000000, -21.77831216351300014 ) ) ;
#9394=DIRECTION ( 'NONE',  ( 0.000000000000000000, 0.000000000000000000, 1.000000000000000000 ) ) ;
#9396=DIRECTION ( 'NONE',  ( 0.000000000000000000, 0.000000000000000000, 1.000000000000000000 ) ) ;
#9397=CARTESIAN_POINT ( 'NONE',  ( 15.50000000000000000, -0.4000000000000000222, -25.99999999999999645 ) ) ;
#9404=ORIENTED_EDGE ( 'NONE', *, *, #9802, .F. ) ;
#9407=PLANE ( 'NONE',  #5366 ) ;
#9408=CARTESIAN_POINT ( 'NONE',  ( 14.25000000000000178, -0.2714405302574884327, 22.98746066354537732 ) ) ;
#9409=ADVANCED_FACE ( 'NONE', ( #8944 ), #15191, .F. ) ;
#9429=CARTESIAN_POINT ( 'NONE',  ( 15.50000000000000000, -0.4000000000000000222, -22.50000000000000000 ) ) ;
#9451=DIRECTION ( 'NONE',  ( 0.000000000000000000, 0.000000000000000000, 1.000000000000000000 ) ) ;
#9463=CARTESIAN_POINT ( 'NONE',  ( -15.50000000000000000, -0.1999999999999999556, 23.94999999999999929 ) ) ;
#9477=CARTESIAN_POINT ( 'NONE',  ( -16.74999999999999289, -0.3152037684892597946, -22.25410949791978510 ) ) ;
#9482=VECTOR ( 'NONE', #6845, 1000.000000000000000 ) ;
#9487=EDGE_CURVE ( 'NONE', #59, #11017, #11923, .T. ) ;
#9492=VECTOR ( 'NONE', #6902, 1000.000000000000000 ) ;
#9509=VERTEX_POINT ( 'NONE', #3066 ) ;
#9510=DIRECTION ( 'NONE',  ( 0.000000000000000000, 1.000000000000000000, 0.000000000000000000 ) ) ;
#9513=ORIENTED_EDGE ( 'NONE', *, *, #1335, .F. ) ;
#9522=EDGE_CURVE ( 'NONE', #9632, #11390, #12385, .T. ) ;
#9564=DIRECTION ( 'NONE',  ( 0.000000000000000000, 0.000000000000000000, 1.000000000000000000 ) ) ;
#9567=ORIENTED_EDGE ( 'NONE', *, *, #5383, .F. ) ;
#9581=DIRECTION ( 'NONE',  ( 0.000000000000000000, 0.000000000000000000, 1.000000000000000000 ) ) ;
#9585=CARTESIAN_POINT ( 'NONE',  ( 23.25000000000000000, -10.00000000000000000, 27.00000000000000000 ) ) ;
#9592=EDGE_LOOP ( 'NONE', ( #14413, #1796, #3417, #2792 ) ) ;
#9597=FACE_OUTER_BOUND ( 'NONE', #3341, .T. ) ;
#9603=CARTESIAN_POINT ( 'NONE',  ( 15.50000000000000000, -0.2000000000000000111, -22.50000000000000000 ) ) ;
#9606=DIRECTION ( 'NONE',  ( 0.000000000000000000, 1.000000000000000000, 0.000000000000000000 ) ) ;
#9608=EDGE_LOOP ( 'NONE', ( #15029, #13640, #9763, #3679 ) ) ;
#9611=ORIENTED_EDGE ( 'NONE', *, *, #7216, .F. ) ;
#9619=LINE ( 'NONE', #14352, #1362 ) ;
#9620=DIRECTION ( 'NONE',  ( -0.9375000000000004441, 0.000000000000000000, -0.3479852726768752902 ) ) ;
#9626=CARTESIAN_POINT ( 'NONE',  ( -14.25000000000000000, -0.2038245569916330158, -21.77831216351300014 ) ) ;
#9627=CARTESIAN_POINT ( 'NONE',  ( -16.75000000000000000, -0.2038245569916330158, -21.77831216351300014 ) ) ;
#9632=VERTEX_POINT ( 'NONE', #4534 ) ;
#9645=CARTESIAN_POINT ( 'NONE',  ( 15.50000000000000000, -1.037157890325000054, 22.50000000000000000 ) ) ;
#9649=ORIENTED_EDGE ( 'NONE', *, *, #11424, .T. ) ;
#9657=ORIENTED_EDGE ( 'NONE', *, *, #4607, .T. ) ;
#9660=EDGE_CURVE ( 'NONE', #215, #5825, #12909, .T. ) ;
#9666=ORIENTED_EDGE ( 'NONE', *, *, #10523, .F. ) ;
#9667=B_SPLINE_CURVE_WITH_KNOTS ( 'NONE', 3,
 ( #3334, #13821, #7916, #8067, #15041, #12883 ),
 .UNSPECIFIED., .F., .F.,
 ( 4, 2, 4 ),
 ( 0.0002380763768129734448, 0.7291065797294589146, 1.457975083082104995 ),
 .UNSPECIFIED. ) ;
#9671=AXIS2_PLACEMENT_3D ( 'NONE', #14566, #4015, #12163 ) ;
#9675=EDGE_CURVE ( 'NONE', #11390, #3042, #8708, .T. ) ;
#9678=EDGE_LOOP ( 'NONE', ( #13030, #5638, #4027, #14272, #4437, #9649 ) ) ;
#9697=ADVANCED_FACE ( 'NONE', ( #15302 ), #5008, .T. ) ;
#9698=CARTESIAN_POINT ( 'NONE',  ( -14.45366306705349224, -0.2717122460102528447, -21.66072723692568402 ) ) ;
#9699=CARTESIAN_POINT ( 'NONE',  ( 16.74999999999999289, -0.3152037684892571301, -22.74589050208021845 ) ) ;
#9705=EDGE_CURVE ( 'NONE', #11017, #6230, #3019, .T. ) ;
#9708=AXIS2_PLACEMENT_3D ( 'NONE', #13064, #10799, #9620 ) ;
#9714=DIRECTION ( 'NONE',  ( 0.000000000000000000, 0.000000000000000000, 1.000000000000000000 ) ) ;
#9754=CARTESIAN_POINT ( 'NONE',  ( 15.08565937784311117, -0.3156604612129180754, -21.29584399676446793 ) ) ;
#9755=CARTESIAN_POINT ( 'NONE',  ( -15.50000000000000000, -0.4000000000005236034, -25.79999999999947136 ) ) ;
#9756=AXIS2_PLACEMENT_3D ( 'NONE', #1228, #13116, #2464 ) ;
#9763=ORIENTED_EDGE ( 'NONE', *, *, #5673, .F. ) ;
#9772=EDGE_CURVE ( 'NONE', #5866, #13359, #12679, .T. ) ;
#9789=EDGE_CURVE ( 'NONE', #5891, #1706, #31, .T. ) ;
#9795=CARTESIAN_POINT ( 'NONE',  ( 15.29686605390242526, -0.2715358723600077018, -23.82609623451301317 ) ) ;
#9798=AXIS2_PLACEMENT_3D ( 'NONE', #3485, #5993, #66 ) ;
#9802=EDGE_CURVE ( 'NONE', #4608, #215, #9941, .T. ) ;
#9804=ORIENTED_EDGE ( 'NONE', *, *, #12867, .T. ) ;
#9809=VECTOR ( 'NONE', #252, 1000.000000000000000 ) ;
#9815=EDGE_CURVE ( 'NONE', #10442, #4229, #2476, .T. ) ;
#9832=ORIENTED_EDGE ( 'NONE', *, *, #5074, .F. ) ;
#9839=DIRECTION ( 'NONE',  ( 0.000000000000000000, 1.000000000000000000, 0.000000000000000000 ) ) ;
#9870=CARTESIAN_POINT ( 'NONE',  ( -23.25000000000000000, -10.00000000000000000, -27.00000000000000000 ) ) ;
#9872=CARTESIAN_POINT ( 'NONE',  ( 14.25000000000000000, -2.500000000000000000, 21.77831216351300014 ) ) ;
#9881=ORIENTED_EDGE ( 'NONE', *, *, #4951, .F. ) ;
#9892=DIRECTION ( 'NONE',  ( 0.000000000000000000, 1.000000000000000000, 0.000000000000000000 ) ) ;
#9899=APPLICATION_CONTEXT ( 'automotive_design' ) ;
#9901=EDGE_CURVE ( 'NONE', #14906, #1551, #11434, .T. ) ;
#9910=FILL_AREA_STYLE_COLOUR ( '', #14907 ) ;
#9912=ADVANCED_FACE ( 'NONE', ( #6187 ), #253, .F. ) ;
#9915=CARTESIAN_POINT ( 'NONE',  ( -15.29686605391142606, -0.2715358723588648937, 23.82609623451821079 ) ) ;
#9925=CARTESIAN_POINT ( 'NONE',  ( -16.75000000000000000, -0.2038245569916330158, 21.77831216351300014 ) ) ;
#9931=CARTESIAN_POINT ( 'NONE',  ( 16.75000000000000000, -0.3156864504677172611, -22.25638000318208398 ) ) ;
#9941=CIRCLE ( 'NONE', #10431, 4.000000000000001776 ) ;
#9946=FACE_BOUND ( 'NONE', #873, .T. ) ;
#9967=DIRECTION ( 'NONE',  ( 0.000000000000000000, -0.000000000000000000, 1.000000000000000000 ) ) ;
#9968=FACE_OUTER_BOUND ( 'NONE', #5032, .T. ) ;
#9984=VECTOR ( 'NONE', #6376, 999.9999999999998863 ) ;
#9986=CARTESIAN_POINT ( 'NONE',  ( -14.25000000000000000, -0.3156864504677185379, -22.25638000318209109 ) ) ;
#10019=ORIENTED_EDGE ( 'NONE', *, *, #14731, .F. ) ;
#10028=CARTESIAN_POINT ( 'NONE',  ( -15.50000000000000000, -0.2038245569916614930, 23.94337567297399971 ) ) ;
#10038=( GEOMETRIC_REPRESENTATION_CONTEXT ( 3 ) GLOBAL_UNCERTAINTY_ASSIGNED_CONTEXT ( ( #11186 ) ) GLOBAL_UNIT_ASSIGNED_CONTEXT ( ( #4631, #12620, #5801 ) ) REPRESENTATION_CONTEXT ( 'NONE', 'WORKASPACE' ) );
#10045=CARTESIAN_POINT ( 'NONE',  ( 15.50000000000000000, -0.2000000000000000111, -19.19999999702029925 ) ) ;
#10048=CARTESIAN_POINT ( 'NONE',  ( -14.25000000000000000, -2.500000000000000000, -21.77831216351300014 ) ) ;
#10050=VECTOR ( 'NONE', #10118, 1000.000000000000114 ) ;
#10052=EDGE_LOOP ( 'NONE', ( #11116, #10905 ) ) ;
#10058=STYLED_ITEM ( 'NONE', ( #475 ), #5426 ) ;
#10076=AXIS2_PLACEMENT_3D ( 'NONE', #7480, #6097, #7405 ) ;
#10078=CARTESIAN_POINT ( 'NONE',  ( 14.24999999999999822, -0.2715193793361447838, -22.98718409945083252 ) ) ;
#10100=CARTESIAN_POINT ( 'NONE',  ( 16.75000000000000000, -2.500000000000000000, -23.22168783648699986 ) ) ;
#10114=DIRECTION ( 'NONE',  ( 0.4999999999999827360, 0.000000000000000000, 0.8660254037844485886 ) ) ;
#10115=CARTESIAN_POINT ( 'NONE',  ( 14.25000000000000000, -0.2038245569916330158, 21.77831216351300014 ) ) ;
#10118=DIRECTION ( 'NONE',  ( -0.8660254037844482555, 0.000000000000000000, -0.4999999999999831801 ) ) ;
#10121=AXIS2_PLACEMENT_3D ( 'NONE', #6726, #6658, #662 ) ;
#10138=ORIENTED_EDGE ( 'NONE', *, *, #997, .F. ) ;
#10142=DIRECTION ( 'NONE',  ( 0.000000000000000000, 1.000000000000000000, 0.000000000000000000 ) ) ;
#10155=LINE ( 'NONE', #6401, #7778 ) ;
#10197=SURFACE_STYLE_FILL_AREA ( #11607 ) ;
#10214=ORIENTED_EDGE ( 'NONE', *, *, #7830, .F. ) ;
#10228=DIRECTION ( 'NONE',  ( 0.8660254037844482555, 0.000000000000000000, 0.4999999999999831801 ) ) ;
#10230=VECTOR ( 'NONE', #9510, 1000.000000000000000 ) ;
#10249=CARTESIAN_POINT ( 'NONE',  ( 15.50000000000000000, 998.9628421096749662, 22.50000000000000000 ) ) ;
#10250=DIRECTION ( 'NONE',  ( 0.000000000000000000, 0.000000000000000000, 1.000000000000000000 ) ) ;
#10251=VERTEX_POINT ( 'NONE', #13975 ) ;
#10252=CARTESIAN_POINT ( 'NONE',  ( 14.45313394609757296, -0.2715358723599912150, 23.33896727494797929 ) ) ;
#10254=CIRCLE ( 'NONE', #11009, 3.499999999999999556 ) ;
#10258=EDGE_CURVE ( 'NONE', #6972, #2946, #8081, .T. ) ;
#10261=VERTEX_POINT ( 'NONE', #10877 ) ;
#10263=EDGE_CURVE ( 'NONE', #14030, #71, #5932, .T. ) ;
#10264=DIRECTION ( 'NONE',  ( 0.000000000000000000, 1.000000000000000000, 0.000000000000000000 ) ) ;
#10269=LINE ( 'NONE', #14999, #3882 ) ;
#10272=EDGE_CURVE ( 'NONE', #7322, #11599, #2416, .T. ) ;
#10273=ORIENTED_EDGE ( 'NONE', *, *, #9487, .T. ) ;
#10274=SURFACE_SIDE_STYLE ('',( #10197 ) ) ;
#10277=AXIS2_PLACEMENT_3D ( 'NONE', #747, #13796, #5505 ) ;
#10279=EDGE_CURVE ( 'NONE', #9632, #1114, #1038, .T. ) ;
#10284=DIRECTION ( 'NONE',  ( 0.000000000000000000, 1.000000000000000000, 0.000000000000000000 ) ) ;
#10290=DIRECTION ( 'NONE',  ( 0.000000000000000000, 1.000000000000000000, 0.000000000000000000 ) ) ;
#10300=VERTEX_POINT ( 'NONE', #9463 ) ;
#10313=CARTESIAN_POINT ( 'NONE',  ( -15.50000000000000000, -1.037157890325000054, -26.00000000000000000 ) ) ;
#10316=AXIS2_PLACEMENT_3D ( 'NONE', #5913, #1229, #1072 ) ;
#10329=DIRECTION ( 'NONE',  ( 0.000000000000000000, 1.000000000000000000, 0.000000000000000000 ) ) ;
#10353=VECTOR ( 'NONE', #5248, 1000.000000000000000 ) ;
#10361=AXIS2_PLACEMENT_3D ( 'NONE', #8028, #6579, #14849 ) ;
#10368=LINE ( 'NONE', #10522, #9492 ) ;
#10399=CYLINDRICAL_SURFACE ( 'NONE', #14796, 4.000000000000000000 ) ;
#10402=VERTEX_POINT ( 'NONE', #1715 ) ;
#10404=ORIENTED_EDGE ( 'NONE', *, *, #5714, .T. ) ;
#10408=EDGE_LOOP ( 'NONE', ( #3739, #1169, #6228, #608 ) ) ;
#10412=DIRECTION ( 'NONE',  ( 0.000000000000000000, -1.000000000000000000, -0.000000000000000000 ) ) ;
#10414=DIRECTION ( 'NONE',  ( 0.4999999999999827360, 0.000000000000000000, 0.8660254037844485886 ) ) ;
#10425=( NAMED_UNIT ( * ) PLANE_ANGLE_UNIT ( ) SI_UNIT ( $, .RADIAN. ) );
#10431=AXIS2_PLACEMENT_3D ( 'NONE', #183, #13310, #13084 ) ;
#10439=PLANE ( 'NONE',  #4551 ) ;
#10442=VERTEX_POINT ( 'NONE', #9300 ) ;
#10453=PLANE ( 'NONE',  #7991 ) ;
#10464=EDGE_CURVE ( 'NONE', #6904, #3116, #2168, .T. ) ;
#10468=ORIENTED_EDGE ( 'NONE', *, *, #1095, .F. ) ;
#10477=CARTESIAN_POINT ( 'NONE',  ( -14.25000000000000178, -0.2714405302574902090, 22.01253933645463690 ) ) ;
#10489=CONICAL_SURFACE ( 'NONE', #2829, 1732.050807568785558, 1.047197551196574761 ) ;
#10497=FACE_BOUND ( 'NONE', #11002, .T. ) ;
#10499=CONICAL_SURFACE ( 'NONE', #93, 1732.050807568785558, 1.047197551196574761 ) ;
#10503=DIRECTION ( 'NONE',  ( 0.000000000000000000, 0.000000000000000000, 1.000000000000000000 ) ) ;
#10506=CARTESIAN_POINT ( 'NONE',  ( -15.29633693294650421, -0.2717122460102743275, 21.17420925361331641 ) ) ;
#10508=EDGE_LOOP ( 'NONE', ( #15091, #14649, #1853, #13622 ) ) ;
#10522=CARTESIAN_POINT ( 'NONE',  ( -15.50000000000000000, -1.037157890325000054, 22.50000000000000000 ) ) ;
#10523=EDGE_CURVE ( 'NONE', #4906, #6230, #6287, .T. ) ;
#10524=ORIENTED_EDGE ( 'NONE', *, *, #14094, .F. ) ;
#10531=MANIFOLD_SOLID_BREP ( 'Cut-Extrude1[5]', #14005 ) ;
#10533=CIRCLE ( 'NONE', #6110, 3.499999999999999556 ) ;
#10534=AXIS2_PLACEMENT_3D ( 'NONE', #7897, #12627, #6741 ) ;
#10545=ORIENTED_EDGE ( 'NONE', *, *, #967, .F. ) ;
#10546=CARTESIAN_POINT ( 'NONE',  ( -15.29633693294650421, -0.2717122460102769921, -23.82579074638668715 ) ) ;
#10547=AXIS2_PLACEMENT_3D ( 'NONE', #314, #2727, #12 ) ;
#10552=VECTOR ( 'NONE', #8964, 1000.000000000000000 ) ;
#10561=DIRECTION ( 'NONE',  ( 0.000000000000000000, 1.000000000000000000, 0.000000000000000000 ) ) ;
#10564=EDGE_CURVE ( 'NONE', #3511, #71, #9152, .T. ) ;
#10566=EDGE_LOOP ( 'NONE', ( #5725, #1511 ) ) ;
#10568=ADVANCED_FACE ( 'NONE', ( #2779 ), #1620, .F. ) ;
#10569=EDGE_LOOP ( 'NONE', ( #2948, #13909 ) ) ;
#10570=ADVANCED_FACE ( 'NONE', ( #14715 ), #1843, .F. ) ;
#10598=DIRECTION ( 'NONE',  ( 0.000000000000000000, 1.000000000000000000, 0.000000000000000000 ) ) ;
#10612=B_SPLINE_CURVE_WITH_KNOTS ( 'NONE', 3,
 ( #12690, #9349, #3384, #8116, #10506, #15235 ),
 .UNSPECIFIED., .F., .F.,
 ( 4, 2, 4 ),
 ( 0.0002380763768132926339, 0.7291065797294586925, 1.457975083082104106 ),
 .UNSPECIFIED. ) ;
#10617=ADVANCED_FACE ( 'NONE', ( #7682 ), #11236, .F. ) ;
#10623=DIRECTION ( 'NONE',  ( 0.000000000000000000, 1.000000000000000000, 0.000000000000000000 ) ) ;
#10626=EDGE_LOOP ( 'NONE', ( #14141, #12092, #6503, #8913 ) ) ;
#10628=ORIENTED_EDGE ( 'NONE', *, *, #6225, .T. ) ;
#10635=FACE_OUTER_BOUND ( 'NONE', #14804, .T. ) ;
#10636=MANIFOLD_SOLID_BREP ( 'Cut-Extrude3', #1340 ) ;
#10637=CARTESIAN_POINT ( 'NONE',  ( -15.91434062215689060, -0.3156604612129251808, 23.70415600323552852 ) ) ;
#10642=ORIENTED_EDGE ( 'NONE', *, *, #4515, .F. ) ;
#10649=EDGE_CURVE ( 'NONE', #1855, #11286, #12204, .T. ) ;
#10652=EDGE_CURVE ( 'NONE', #6972, #2099, #3542, .T. ) ;
#10654=CARTESIAN_POINT ( 'NONE',  ( 15.50000000000000000, 0.000000000000000000, -22.50000000000000000 ) ) ;
#10685=ORIENTED_EDGE ( 'NONE', *, *, #13714, .F. ) ;
#10686=VECTOR ( 'NONE', #10264, 1000.000000000000000 ) ;
#10697=CARTESIAN_POINT ( 'NONE',  ( 14.25000000000000000, -2.500000000000000000, -21.77831216351300014 ) ) ;
#10705=AXIS2_PLACEMENT_3D ( 'NONE', #7859, #13894, #3198 ) ;
#10711=VECTOR ( 'NONE', #3466, 1000.000000000000114 ) ;
#10715=CARTESIAN_POINT ( 'NONE',  ( 15.50000000000000000, -2.500000000000000000, -21.05662432702600029 ) ) ;
#10723=VERTEX_POINT ( 'NONE', #14018 ) ;
#10737=AXIS2_PLACEMENT_3D ( 'NONE', #3821, #8547, #6399 ) ;
#10778=DIRECTION ( 'NONE',  ( 0.000000000000000000, 1.000000000000000000, 0.000000000000000000 ) ) ;
#10782=( NAMED_UNIT ( * ) PLANE_ANGLE_UNIT ( ) SI_UNIT ( $, .RADIAN. ) );
#10789=CARTESIAN_POINT ( 'NONE',  ( -15.50000000000000000, -2.500000000000000000, -21.05662432702600029 ) ) ;
#10799=DIRECTION ( 'NONE',  ( 0.000000000000000000, 1.000000000000000000, 0.000000000000000000 ) ) ;
#10802=CARTESIAN_POINT ( 'NONE',  ( -16.54686605390243059, -0.2715358723599923807, 23.33896727494797929 ) ) ;
#10803=DIRECTION ( 'NONE',  ( 0.000000000000000000, 1.000000000000000000, 0.000000000000000000 ) ) ;
#10804=CIRCLE ( 'NONE', #10547, 3.499999999999999556 ) ;
#10805=DIRECTION ( 'NONE',  ( 0.000000000000000000, 1.000000000000000000, 0.000000000000000000 ) ) ;
#10813=CARTESIAN_POINT ( 'NONE',  ( -15.50000000000000000, -0.4000000000000000222, -22.50000000000000000 ) ) ;
#10835=ADVANCED_FACE ( 'NONE', ( #122 ), #4876, .F. ) ;
#10847=EDGE_LOOP ( 'NONE', ( #3525, #13279, #1424, #13343 ) ) ;
#10860=ADVANCED_FACE ( 'NONE', ( #736 ), #5249, .F. ) ;
#10862=( LENGTH_UNIT ( ) NAMED_UNIT ( * ) SI_UNIT ( .MILLI., .METRE. ) );
#10871=ORIENTED_EDGE ( 'NONE', *, *, #4951, .T. ) ;
#10877=CARTESIAN_POINT ( 'NONE',  ( -15.50000000000000000, -2.500000000000000000, -21.05662432702600029 ) ) ;
#10882=CARTESIAN_POINT ( 'NONE',  ( -15.70366306705060033, -0.2717122460100995229, 23.82579074638835692 ) ) ;
#10896=CARTESIAN_POINT ( 'NONE',  ( 15.50000000000000000, -1.037157890325000054, -22.50000000000000000 ) ) ;
#10897=DIRECTION ( 'NONE',  ( 0.000000000000000000, 1.000000000000000000, 0.000000000000000000 ) ) ;
#10905=ORIENTED_EDGE ( 'NONE', *, *, #4389, .T. ) ;
#10927=CARTESIAN_POINT ( 'NONE',  ( -15.50000000000000000, -0.2000000000000000111, -22.50000000000000000 ) ) ;
#10929=CIRCLE ( 'NONE', #9671, 1.449999999999999956 ) ;
#10960=ORIENTED_EDGE ( 'NONE', *, *, #12162, .F. ) ;
#10978=AXIS2_PLACEMENT_3D ( 'NONE', #5603, #3329, #11788 ) ;
#10998=VERTEX_POINT ( 'NONE', #6934 ) ;
#11002=EDGE_LOOP ( 'NONE', ( #4374, #12035 ) ) ;
#11007=CARTESIAN_POINT ( 'NONE',  ( 15.50000000000000000, -5.000000000000000000, 18.50000000000000000 ) ) ;
#11009=AXIS2_PLACEMENT_3D ( 'NONE', #7463, #14581, #4037 ) ;
#11011=AXIS2_PLACEMENT_3D ( 'NONE', #6093, #10805, #3504 ) ;
#11017=VERTEX_POINT ( 'NONE', #9397 ) ;
#11021=TOROIDAL_SURFACE ( 'NONE', #11011, 3.299999999999470024, 0.2000000000005275058 ) ;
#11023=CIRCLE ( 'NONE', #4336, 0.2000000000005226763 ) ;
#11029=LINE ( 'NONE', #14431, #13725 ) ;
#11033=ORIENTED_EDGE ( 'NONE', *, *, #6501, .T. ) ;
#11035=COLOUR_RGB ( '', 0.66274510, 0.83137255, 0.94901961) ;
#11040=VECTOR ( 'NONE', #7634, 1000.000000000000000 ) ;
#11045=CARTESIAN_POINT ( 'NONE',  ( -15.50000000000000000, -1.037157890325000054, -22.50000000000000000 ) ) ;
#11049=CARTESIAN_POINT ( 'NONE',  ( -15.50000000000000000, -0.4000000000005236034, -22.50000000000000000 ) ) ;
#11050=AXIS2_PLACEMENT_3D ( 'NONE', #6946, #10414, #12761 ) ;
#11051=DIRECTION ( 'NONE',  ( 0.000000000000000000, 0.000000000000000000, 1.000000000000000000 ) ) ;
#11057=ORIENTED_EDGE ( 'NONE', *, *, #6320, .T. ) ;
#11060=EDGE_LOOP ( 'NONE', ( #8046, #4465, #13281, #4581 ) ) ;
#11072=B_SPLINE_CURVE_WITH_KNOTS ( 'NONE', 3,
 ( #8871, #9795, #8710, #12292, #8562, #4148 ),
 .UNSPECIFIED., .F., .F.,
 ( 4, 2, 4 ),
 ( 0.0002380763768130567115, 0.7291065797294590256, 1.457975083082104995 ),
 .UNSPECIFIED. ) ;
#11090=DIRECTION ( 'NONE',  ( 0.000000000000000000, 0.000000000000000000, -1.000000000000000000 ) ) ;
#11104=FACE_OUTER_BOUND ( 'NONE', #1150, .T. ) ;
#11107=DIRECTION ( 'NONE',  ( 0.000000000000000000, 0.000000000000000000, 1.000000000000000000 ) ) ;
#11111=VERTEX_POINT ( 'NONE', #6014 ) ;
#11114=VECTOR ( 'NONE', #6051, 1000.000000000000000 ) ;
#11116=ORIENTED_EDGE ( 'NONE', *, *, #7727, .T. ) ;
#11121=EDGE_CURVE ( 'NONE', #11427, #3938, #11966, .T. ) ;
#11124=CARTESIAN_POINT ( 'NONE',  ( 15.50000000000000000, -0.2000000000000000111, -25.80000000297970075 ) ) ;
#11138=DIRECTION ( 'NONE',  ( 0.000000000000000000, 1.000000000000000000, 0.000000000000000000 ) ) ;
#11152=ADVANCED_FACE ( 'NONE', ( #12275 ), #2572, .T. ) ;
#11153=ADVANCED_FACE ( 'NONE', ( #8624 ), #5149, .F. ) ;
#11159=CARTESIAN_POINT ( 'NONE',  ( -14.25000000000000000, -0.2038245569916330158, -23.22168783648699986 ) ) ;
#11160=LINE ( 'NONE', #5275, #12011 ) ;
#11166=VERTEX_POINT ( 'NONE', #9627 ) ;
#11167=ORIENTED_EDGE ( 'NONE', *, *, #6216, .F. ) ;
#11185=EDGE_LOOP ( 'NONE', ( #915, #523, #14420, #14107, #14154, #6700 ) ) ;
#11186=UNCERTAINTY_MEASURE_WITH_UNIT (LENGTH_MEASURE( 1.000000000000000082E-05 ), #4631, 'distance_accuracy_value', 'NONE');
#11189=VECTOR ( 'NONE', #6799, 999.9999999999998863 ) ;
#11195=VECTOR ( 'NONE', #1141, 1000.000000000000000 ) ;
#11200=EDGE_CURVE ( 'NONE', #7389, #6830, #12846, .T. ) ;
#11209=( GEOMETRIC_REPRESENTATION_CONTEXT ( 3 ) GLOBAL_UNCERTAINTY_ASSIGNED_CONTEXT ( ( #2815 ) ) GLOBAL_UNIT_ASSIGNED_CONTEXT ( ( #7825, #5272, #6897 ) ) REPRESENTATION_CONTEXT ( 'NONE', 'WORKASPACE' ) );
#11225=ORIENTED_EDGE ( 'NONE', *, *, #1161, .F. ) ;
#11236=PLANE ( 'NONE',  #14173 ) ;
#11238=EDGE_CURVE ( 'NONE', #1706, #13129, #7988, .T. ) ;
#11240=EDGE_CURVE ( 'NONE', #4720, #3939, #11910, .T. ) ;
#11242=DIRECTION ( 'NONE',  ( 0.8660254037844482555, 0.000000000000000000, -0.4999999999999831801 ) ) ;
#11243=AXIS2_PLACEMENT_3D ( 'NONE', #6396, #2489, #11107 ) ;
#11244=VECTOR ( 'NONE', #2477, 1000.000000000000000 ) ;
#11249=ORIENTED_EDGE ( 'NONE', *, *, #11238, .F. ) ;
#11257=CARTESIAN_POINT ( 'NONE',  ( 15.50000000000000000, -5.000000000000000000, 26.00000000000000000 ) ) ;
#11272=CARTESIAN_POINT ( 'NONE',  ( -14.25000000000000000, -2.500000000000000000, 23.22168783648699986 ) ) ;
#11286=VERTEX_POINT ( 'NONE', #6545 ) ;
#11297=CARTESIAN_POINT ( 'NONE',  ( -14.25000000000000000, -2.500000000000000000, -21.77831216351300014 ) ) ;
#11306=VECTOR ( 'NONE', #2341, 1000.000000000000000 ) ;
#11331=CIRCLE ( 'NONE', #9342, 3.299999999999473577 ) ;
#11337=EDGE_CURVE ( 'NONE', #11166, #13163, #8582, .T. ) ;
#11341=ORIENTED_EDGE ( 'NONE', *, *, #7465, .F. ) ;
#11345=CIRCLE ( 'NONE', #1681, 4.000000000000000000 ) ;
#11359=ORIENTED_EDGE ( 'NONE', *, *, #1916, .T. ) ;
#11374=DIRECTION ( 'NONE',  ( 0.000000000000000000, 0.000000000000000000, 1.000000000000000000 ) ) ;
#11377=DIRECTION ( 'NONE',  ( 0.000000000000000000, 1.000000000000000000, 0.000000000000000000 ) ) ;
#11379=DIRECTION ( 'NONE',  ( 0.000000000000000000, 0.000000000000000000, 1.000000000000000000 ) ) ;
#11385=FACE_OUTER_BOUND ( 'NONE', #10626, .T. ) ;
#11387=ORIENTED_EDGE ( 'NONE', *, *, #799, .T. ) ;
#11388=VERTEX_POINT ( 'NONE', #9381 ) ;
#11390=VERTEX_POINT ( 'NONE', #7074 ) ;
#11401=DIRECTION ( 'NONE',  ( 0.000000000000000000, 1.000000000000000000, 0.000000000000000000 ) ) ;
#11409=ORIENTED_EDGE ( 'NONE', *, *, #11826, .T. ) ;
#11423=LINE ( 'NONE', #4522, #14479 ) ;
#11424=EDGE_CURVE ( 'NONE', #10300, #777, #7035, .T. ) ;
#11427=VERTEX_POINT ( 'NONE', #6919 ) ;
#11434=CIRCLE ( 'NONE', #13183, 3.300000002979700753 ) ;
#11441=DIRECTION ( 'NONE',  ( 0.000000000000000000, 0.000000000000000000, 1.000000000000000000 ) ) ;
#11460=PLANE ( 'NONE',  #593 ) ;
#11491=ORIENTED_EDGE ( 'NONE', *, *, #1112, .T. ) ;
#11500=CARTESIAN_POINT ( 'NONE',  ( -14.25000000000000000, -2.500000000000000000, -21.77831216351300014 ) ) ;
#11520=DIRECTION ( 'NONE',  ( 0.000000000000000000, 1.000000000000000000, 0.000000000000000000 ) ) ;
#11528=ORIENTED_EDGE ( 'NONE', *, *, #6225, .F. ) ;
#11542=AXIS2_PLACEMENT_3D ( 'NONE', #2610, #9892, #14620 ) ;
#11563=CIRCLE ( 'NONE', #8598, 3.499999999999999556 ) ;
#11564=FACE_OUTER_BOUND ( 'NONE', #5208, .T. ) ;
#11569=CARTESIAN_POINT ( 'NONE',  ( -15.50000000000000000, -2.500000000000000000, 21.05662432702600029 ) ) ;
#11573=EDGE_CURVE ( 'NONE', #3973, #9306, #13354, .T. ) ;
#11582=FACE_OUTER_BOUND ( 'NONE', #1009, .T. ) ;
#11591=EDGE_CURVE ( 'NONE', #4688, #11111, #14572, .T. ) ;
#11595=DIRECTION ( 'NONE',  ( 0.000000000000000000, 0.000000000000000000, 1.000000000000000000 ) ) ;
#11596=CARTESIAN_POINT ( 'NONE',  ( -15.50000000000000000, 998.9628421096749662, 22.50000000000000000 ) ) ;
#11599=VERTEX_POINT ( 'NONE', #12171 ) ;
#11607=FILL_AREA_STYLE ('',( #4395 ) ) ;
#11611=FACE_OUTER_BOUND ( 'NONE', #15174, .T. ) ;
#11618=CARTESIAN_POINT ( 'NONE',  ( -14.25000000000000000, -2.500000000000000000, -23.22168783648699986 ) ) ;
#11621=CARTESIAN_POINT ( 'NONE',  ( 23.25000000000000000, -5.000000000000000000, -27.00000000000000000 ) ) ;
#11639=ORIENTED_EDGE ( 'NONE', *, *, #15221, .F. ) ;
#11640=CARTESIAN_POINT ( 'NONE',  ( -15.08565937784311295, -0.3156604612129216836, -23.70415600323552852 ) ) ;
#11645=CARTESIAN_POINT ( 'NONE',  ( -16.75000000000000000, -0.2038245569916330158, -23.22168783648699986 ) ) ;
#11648=DIRECTION ( 'NONE',  ( 0.000000000000000000, 0.000000000000000000, 1.000000000000000000 ) ) ;
#11652=CARTESIAN_POINT ( 'NONE',  ( -30.00000000000000000, 0.000000000000000000, 27.00000000000000000 ) ) ;
#11663=DIRECTION ( 'NONE',  ( 0.000000000000000000, 1.000000000000000000, 0.000000000000000000 ) ) ;
#11664=ADVANCED_FACE ( 'NONE', ( #150 ), #6300, .T. ) ;
#11668=EDGE_CURVE ( 'NONE', #5825, #5722, #8036, .T. ) ;
#11676=PRESENTATION_STYLE_ASSIGNMENT (( #13854 ) ) ;
#11684=DIRECTION ( 'NONE',  ( -0.9375000000000004441, 0.000000000000000000, -0.3479852726768752902 ) ) ;
#11689=CIRCLE ( 'NONE', #8715, 3.300000002979700753 ) ;
#11693=DIRECTION ( 'NONE',  ( 0.000000000000000000, 1.000000000000000000, 0.000000000000000000 ) ) ;
#11699=EDGE_LOOP ( 'NONE', ( #13175, #15327, #8945, #15139 ) ) ;
#11700=ORIENTED_EDGE ( 'NONE', *, *, #4204, .T. ) ;
#11706=DIRECTION ( 'NONE',  ( 0.000000000000000000, 0.000000000000000000, 1.000000000000000000 ) ) ;
#11715=CARTESIAN_POINT ( 'NONE',  ( 14.25000000000000000, -2.500000000000000000, -23.22168783648699986 ) ) ;
#11721=ORIENTED_EDGE ( 'NONE', *, *, #10464, .T. ) ;
#11722=EDGE_CURVE ( 'NONE', #7228, #8110, #8834, .T. ) ;
#11728=EDGE_CURVE ( 'NONE', #10442, #777, #11160, .T. ) ;
#11741=EDGE_LOOP ( 'NONE', ( #9404, #14912, #13635, #3386 ) ) ;
#11744=ORIENTED_EDGE ( 'NONE', *, *, #11955, .T. ) ;
#11745=AXIS2_PLACEMENT_3D ( 'NONE', #12257, #12488, #8909 ) ;
#11753=VECTOR ( 'NONE', #7052, 1000.000000000000000 ) ;
#11755=ORIENTED_EDGE ( 'NONE', *, *, #12184, .T. ) ;
#11786=AXIS2_PLACEMENT_3D ( 'NONE', #9755, #12250, #11090 ) ;
#11787=PLANE ( 'NONE',  #10316 ) ;
#11788=DIRECTION ( 'NONE',  ( 0.000000000000000000, 0.000000000000000000, 1.000000000000000000 ) ) ;
#11802=EDGE_LOOP ( 'NONE', ( #13344, #5764 ) ) ;
#11819=ADVANCED_FACE ( 'NONE', ( #13722 ), #14795, .F. ) ;
#11826=EDGE_CURVE ( 'NONE', #9509, #6831, #12680, .T. ) ;
#11827=ORIENTED_EDGE ( 'NONE', *, *, #13892, .F. ) ;
#11830=CARTESIAN_POINT ( 'NONE',  ( 15.50000000000000000, 998.9628421096749662, -22.50000000000000000 ) ) ;
#11831=CARTESIAN_POINT ( 'NONE',  ( 14.24999999999999822, -0.3152037684892576297, 22.74589050208021845 ) ) ;
#11864=FACE_OUTER_BOUND ( 'NONE', #4780, .T. ) ;
#11866=EDGE_CURVE ( 'NONE', #11017, #59, #3509, .T. ) ;
#11884=PRODUCT_DEFINITION_FORMATION_WITH_SPECIFIED_SOURCE ( 'ANY', '', #5345, .NOT_KNOWN. ) ;
#11887=PLANE ( 'NONE',  #13499 ) ;
#11889=B_SPLINE_CURVE_WITH_KNOTS ( 'NONE', 3,
 ( #10115, #12540, #1904, #11831, #9408, #26 ),
 .UNSPECIFIED., .F., .F.,
 ( 4, 2, 4 ),
 ( 1.820537833122031657, 2.555393473688636341, 3.290249114255240581 ),
 .UNSPECIFIED. ) ;
#11904=FACE_OUTER_BOUND ( 'NONE', #1850, .T. ) ;
#11906=ADVANCED_FACE ( 'NONE', ( #6823 ), #1217, .F. ) ;
#11910=B_SPLINE_CURVE_WITH_KNOTS ( 'NONE', 3,
 ( #4205, #1871, #6695, #13599, #770, #13745 ),
 .UNSPECIFIED., .F., .F.,
 ( 4, 2, 4 ),
 ( 1.820537833122030991, 2.555393473688635453, 3.290249114255240137 ),
 .UNSPECIFIED. ) ;
#11913=VERTEX_POINT ( 'NONE', #11621 ) ;
#11920=ADVANCED_FACE ( 'NONE', ( #2380 ), #13938, .T. ) ;
#11923=CIRCLE ( 'NONE', #2745, 3.499999999999999556 ) ;
#11953=DIRECTION ( 'NONE',  ( 0.000000000000000000, 0.000000000000000000, -1.000000000000000000 ) ) ;
#11955=EDGE_CURVE ( 'NONE', #4275, #5866, #3468, .T. ) ;
#11956=STYLED_ITEM ( 'NONE', ( #14861 ), #10636 ) ;
#11957=SURFACE_STYLE_USAGE ( .BOTH. , #8079 ) ;
#11963=CARTESIAN_POINT ( 'NONE',  ( -15.50000000000000000, -1.037157890325000054, -22.50000000000000000 ) ) ;
#11966=LINE ( 'NONE', #1332, #6045 ) ;
#11969=ORIENTED_EDGE ( 'NONE', *, *, #14095, .F. ) ;
#11971=ORIENTED_EDGE ( 'NONE', *, *, #4136, .T. ) ;
#11972=CARTESIAN_POINT ( 'NONE',  ( -16.75000000000000000, -2.500000000000000000, 21.77831216351300014 ) ) ;
#11981=CARTESIAN_POINT ( 'NONE',  ( -15.70313394609756585, -0.2715358723600081459, 21.17390376548697262 ) ) ;
#11998=ADVANCED_FACE ( 'NONE', ( #15324 ), #273, .F. ) ;
#12008=DIRECTION ( 'NONE',  ( 0.000000000000000000, 1.000000000000000000, 0.000000000000000000 ) ) ;
#12011=VECTOR ( 'NONE', #4107, 1000.000000000000000 ) ;
#12017=ORIENTED_EDGE ( 'NONE', *, *, #1937, .T. ) ;
#12021=B_SPLINE_CURVE_WITH_KNOTS ( 'NONE', 3,
 ( #6298, #3795, #9986, #14716, #5200, #11159 ),
 .UNSPECIFIED., .F., .F.,
 ( 4, 2, 4 ),
 ( 1.820537833122031213, 2.555393473688635453, 3.290249114255239693 ),
 .UNSPECIFIED. ) ;
#12026=CIRCLE ( 'NONE', #6100, 4.000000000000000888 ) ;
#12035=ORIENTED_EDGE ( 'NONE', *, *, #7465, .T. ) ;
#12044=DIRECTION ( 'NONE',  ( 0.8660254037844485886, 0.000000000000000000, -0.4999999999999827360 ) ) ;
#12045=CARTESIAN_POINT ( 'NONE',  ( -15.50000000000000000, -0.2038245569916614930, 23.94337567297399971 ) ) ;
#12048=DIRECTION ( 'NONE',  ( 1.060575238724893480E-16, 0.5000000000000189848, -0.8660254037844277164 ) ) ;
#12052=ORIENTED_EDGE ( 'NONE', *, *, #3984, .T. ) ;
#12059=AXIS2_PLACEMENT_3D ( 'NONE', #2612, #203, #446 ) ;
#12071=AXIS2_PLACEMENT_3D ( 'NONE', #5962, #966, #15076 ) ;
#12076=CARTESIAN_POINT ( 'NONE',  ( -15.50000000000000000, -0.4000000000000000222, 19.00000000000000355 ) ) ;
#12078=ORIENTED_EDGE ( 'NONE', *, *, #214, .F. ) ;
#12085=DIRECTION ( 'NONE',  ( 0.000000000000000000, 1.000000000000000000, 0.000000000000000000 ) ) ;
#12092=ORIENTED_EDGE ( 'NONE', *, *, #2143, .F. ) ;
#12103=DIRECTION ( 'NONE',  ( 0.000000000000000000, 0.000000000000000000, 1.000000000000000000 ) ) ;
#12105=DIRECTION ( 'NONE',  ( 0.000000000000000000, 0.000000000000000000, 1.000000000000000000 ) ) ;
#12116=CARTESIAN_POINT ( 'NONE',  ( 15.50000000000000000, -2.500000000000000000, -23.94337567297399971 ) ) ;
#12126=DIRECTION ( 'NONE',  ( 0.000000000000000000, 0.000000000000000000, 1.000000000000000000 ) ) ;
#12131=ORIENTED_EDGE ( 'NONE', *, *, #3459, .F. ) ;
#12135=DIRECTION ( 'NONE',  ( 0.000000000000000000, 0.000000000000000000, 1.000000000000000000 ) ) ;
#12148=ADVANCED_FACE ( 'NONE', ( #14783 ), #14701, .F. ) ;
#12152=FACE_OUTER_BOUND ( 'NONE', #5516, .T. ) ;
#12153=DIRECTION ( 'NONE',  ( -0.000000000000000000, 1.000000000000000000, 0.000000000000000000 ) ) ;
#12157=CARTESIAN_POINT ( 'NONE',  ( 15.50000000000000000, -0.2038245569916604938, -21.05662432702600029 ) ) ;
#12161=ORIENTED_EDGE ( 'NONE', *, *, #595, .T. ) ;
#12162=EDGE_CURVE ( 'NONE', #1551, #14906, #11689, .T. ) ;
#12163=DIRECTION ( 'NONE',  ( 0.000000000000000000, 0.000000000000000000, 1.000000000000000000 ) ) ;
#12170=CARTESIAN_POINT ( 'NONE',  ( -15.50000000000000000, -0.4000000000005236034, 22.50000000000000000 ) ) ;
#12171=CARTESIAN_POINT ( 'NONE',  ( 15.50000000000000000, -2.500000000000000000, -23.94337567297399971 ) ) ;
#12173=EDGE_LOOP ( 'NONE', ( #6282, #1476, #8989, #96 ) ) ;
#12184=EDGE_CURVE ( 'NONE', #181, #14839, #1829, .T. ) ;
#12201=ORIENTED_EDGE ( 'NONE', *, *, #3843, .F. ) ;
#12204=CIRCLE ( 'NONE', #8728, 1.449999999999999956 ) ;
#12209=AXIS2_PLACEMENT_3D ( 'NONE', #12920, #5886, #3381 ) ;
#12227=CARTESIAN_POINT ( 'NONE',  ( 15.50000000000000000, -5.000000000000000000, -22.50000000000000000 ) ) ;
#12234=B_SPLINE_CURVE_WITH_KNOTS ( 'NONE', 3,
 ( #1771, #9915, #6302, #4254, #7536, #5279 ),
 .UNSPECIFIED., .F., .F.,
 ( 4, 2, 4 ),
 ( 0.0002380763768129734448, 0.7291065797294585815, 1.457975083082104328 ),
 .UNSPECIFIED. ) ;
#12236=EDGE_LOOP ( 'NONE', ( #14342, #7250, #13648, #14854, #14558, #650 ) ) ;
#12237=ORIENTED_EDGE ( 'NONE', *, *, #11337, .T. ) ;
#12240=LINE ( 'NONE', #5190, #6083 ) ;
#12248=DIRECTION ( 'NONE',  ( -0.000000000000000000, 1.000000000000000000, -0.000000000000000000 ) ) ;
#12250=DIRECTION ( 'NONE',  ( 1.000000000000000000, -0.000000000000000000, 1.224646799147353207E-16 ) ) ;
#12254=VECTOR ( 'NONE', #6933, 1000.000000000000000 ) ;
#12257=CARTESIAN_POINT ( 'NONE',  ( -30.00000000000000000, -5.000000000000000000, -43.00000000000002132 ) ) ;
#12275=FACE_OUTER_BOUND ( 'NONE', #5925, .T. ) ;
#12285=PRODUCT_DEFINITION_CONTEXT ( 'detailed design', #9899, 'design' ) ;
#12288=ADVANCED_FACE ( 'NONE', ( #2060 ), #5532, .F. ) ;
#12292=CARTESIAN_POINT ( 'NONE',  ( 14.66434062215688883, -0.3156604612129108589, -23.46090750622545684 ) ) ;
#12295=CARTESIAN_POINT ( 'NONE',  ( 14.25000000000000000, -2.500000000000000000, 23.22168783648699986 ) ) ;
#12297=EDGE_CURVE ( 'NONE', #3822, #3973, #6809, .T. ) ;
#12300=CARTESIAN_POINT ( 'NONE',  ( 15.50000000000000000, -0.4000000000005274892, 22.50000000000000000 ) ) ;
#12302=ADVANCED_FACE ( 'NONE', ( #14085 ), #12848, .T. ) ;
#12319=CARTESIAN_POINT ( 'NONE',  ( 15.50000000000000000, -1.037157890325000054, 26.00000000000000000 ) ) ;
#12322=EDGE_LOOP ( 'NONE', ( #8230, #3207 ) ) ;
#12329=DIRECTION ( 'NONE',  ( 0.8660254037844482555, 0.000000000000000000, 0.4999999999999831801 ) ) ;
#12332=SURFACE_STYLE_USAGE ( .BOTH. , #5199 ) ;
#12337=CARTESIAN_POINT ( 'NONE',  ( 15.50000000000000000, -0.2038245569916610489, -23.94337567297399971 ) ) ;
#12349=CARTESIAN_POINT ( 'NONE',  ( 14.25000000000000000, -0.3156864504677152627, -22.74361999681790536 ) ) ;
#12351=CARTESIAN_POINT ( 'NONE',  ( 15.91434062215687284, -0.3156604612129197962, 21.29584399676445727 ) ) ;
#12354=CARTESIAN_POINT ( 'NONE',  ( 15.50000000000000000, -0.2038245569916610489, 21.05662432702600029 ) ) ;
#12367=ADVANCED_FACE ( 'NONE', ( #891 ), #7977, .F. ) ;
#12377=CARTESIAN_POINT ( 'NONE',  ( 14.66242688423474583, -0.3152598339554803508, 23.45980260912095616 ) ) ;
#12380=ORIENTED_EDGE ( 'NONE', *, *, #12162, .T. ) ;
#12385=LINE ( 'NONE', #1678, #1512 ) ;
#12388=EDGE_CURVE ( 'NONE', #1628, #4275, #109, .T. ) ;
#12393=CARTESIAN_POINT ( 'NONE',  ( -15.50000000000000000, -0.2000000000000000111, -25.79999999999947136 ) ) ;
#12398=CARTESIAN_POINT ( 'NONE',  ( -15.50000000000000000, -5.000000000000000000, -18.50000000000000000 ) ) ;
#12410=DIRECTION ( 'NONE',  ( 0.000000000000000000, 0.000000000000000000, 1.000000000000000000 ) ) ;
#12435=DIRECTION ( 'NONE',  ( 0.000000000000000000, 0.000000000000000000, -1.000000000000000000 ) ) ;
#12463=CARTESIAN_POINT ( 'NONE',  ( 16.75000000000000000, -2.500000000000000000, 21.77831216351300014 ) ) ;
#12466=EDGE_CURVE ( 'NONE', #3938, #3097, #12657, .T. ) ;
#12469=ORIENTED_EDGE ( 'NONE', *, *, #4097, .T. ) ;
#12483=DIRECTION ( 'NONE',  ( 0.000000000000000000, 0.000000000000000000, 1.000000000000000000 ) ) ;
#12488=DIRECTION ( 'NONE',  ( -0.000000000000000000, 1.000000000000000000, 0.000000000000000000 ) ) ;
#12495=ORIENTED_EDGE ( 'NONE', *, *, #4389, .F. ) ;
#12505=CARTESIAN_POINT ( 'NONE',  ( -16.75000000000000000, -0.2714405302574894319, 22.98746066354538087 ) ) ;
#12506=CARTESIAN_POINT ( 'NONE',  ( -16.75000000000000000, -2.500000000000000000, -23.22168783648699986 ) ) ;
#12510=DIRECTION ( 'NONE',  ( -1.000000000000000000, 0.000000000000000000, 0.000000000000000000 ) ) ;
#12512=ORIENTED_EDGE ( 'NONE', *, *, #1937, .F. ) ;
#12540=CARTESIAN_POINT ( 'NONE',  ( 14.24999999999999822, -0.2715193793361405095, 22.01281590054915327 ) ) ;
#12543=CARTESIAN_POINT ( 'NONE',  ( -30.00000000000000000, -5.000000000000000000, -43.00000000000002132 ) ) ;
#12545=AXIS2_PLACEMENT_3D ( 'NONE', #552, #5380, #5299 ) ;
#12546=CARTESIAN_POINT ( 'NONE',  ( 15.50000000000000000, -5.000000000000000000, -26.50000000000000000 ) ) ;
#12554=VECTOR ( 'NONE', #5491, 1000.000000000000000 ) ;
#12568=EDGE_CURVE ( 'NONE', #11388, #10261, #1246, .T. ) ;
#12579=CARTESIAN_POINT ( 'NONE',  ( 14.25000000000000000, -0.2038245569916330158, -23.22168783648699986 ) ) ;
#12582=AXIS2_PLACEMENT_3D ( 'NONE', #14680, #8872, #11051 ) ;
#12590=ORIENTED_EDGE ( 'NONE', *, *, #10464, .F. ) ;
#12600=DIRECTION ( 'NONE',  ( 0.000000000000000000, 1.000000000000000000, 0.000000000000000000 ) ) ;
#12601=CIRCLE ( 'NONE', #5928, 3.299999999999473577 ) ;
#12613=FACE_OUTER_BOUND ( 'NONE', #14687, .T. ) ;
#12617=CARTESIAN_POINT ( 'NONE',  ( -15.50000000000000000, -5.000000000000000000, -22.50000000000000000 ) ) ;
#12620=( NAMED_UNIT ( * ) PLANE_ANGLE_UNIT ( ) SI_UNIT ( $, .RADIAN. ) );
#12627=DIRECTION ( 'NONE',  ( 0.000000000000000000, 1.000000000000000000, 0.000000000000000000 ) ) ;
#12636=ORIENTED_EDGE ( 'NONE', *, *, #5474, .T. ) ;
#12640=FACE_BOUND ( 'NONE', #10566, .T. ) ;
#12657=B_SPLINE_CURVE_WITH_KNOTS ( 'NONE', 3,
 ( #1099, #3499, #7090, #7164, #10477, #5624 ),
 .UNSPECIFIED., .F., .F.,
 ( 4, 2, 4 ),
 ( 1.820537833122031213, 2.555393473688635453, 3.290249114255239693 ),
 .UNSPECIFIED. ) ;
#12658=CARTESIAN_POINT ( 'NONE',  ( 15.70313394608857394, -0.2715358723588625622, 23.82609623451821079 ) ) ;
#12670=EDGE_CURVE ( 'NONE', #13195, #3511, #1885, .T. ) ;
#12679=LINE ( 'NONE', #2053, #11189 ) ;
#12680=CIRCLE ( 'NONE', #1540, 1.449999999999996403 ) ;
#12683=VECTOR ( 'NONE', #3730, 1000.000000000000114 ) ;
#12690=CARTESIAN_POINT ( 'NONE',  ( -14.25000000000000000, -0.2038245569916330158, 21.77831216351300014 ) ) ;
#12693=AXIS2_PLACEMENT_3D ( 'NONE', #10697, #2470, #5353 ) ;
#12696=AXIS2_PLACEMENT_3D ( 'NONE', #3998, #11138, #13328 ) ;
#12697=CARTESIAN_POINT ( 'NONE',  ( -15.50000000000000000, -0.1999999999999999556, 22.50000000000000000 ) ) ;
#12702=AXIS2_PLACEMENT_3D ( 'NONE', #4986, #3899, #12126 ) ;
#12722=LINE ( 'NONE', #5527, #15228 ) ;
#12729=CARTESIAN_POINT ( 'NONE',  ( 15.50000000000000000, -1.037157890325000054, -26.00000000000000000 ) ) ;
#12730=EDGE_LOOP ( 'NONE', ( #7460, #14497 ) ) ;
#12732=EDGE_LOOP ( 'NONE', ( #9881, #14802, #5977, #2965 ) ) ;
#12740=EDGE_CURVE ( 'NONE', #7739, #9509, #9074, .T. ) ;
#12753=VERTEX_POINT ( 'NONE', #7772 ) ;
#12754=EDGE_CURVE ( 'NONE', #4229, #3116, #8375, .T. ) ;
#12761=DIRECTION ( 'NONE',  ( 0.8660254037844485886, 0.000000000000000000, -0.4999999999999827360 ) ) ;
#12768=DIRECTION ( 'NONE',  ( 0.000000000000000000, 0.000000000000000000, 1.000000000000000000 ) ) ;
#12780=AXIS2_PLACEMENT_3D ( 'NONE', #3067, #10114, #9176 ) ;
#12788=ORIENTED_EDGE ( 'NONE', *, *, #14094, .T. ) ;
#12809=ORIENTED_EDGE ( 'NONE', *, *, #6895, .F. ) ;
#12813=CARTESIAN_POINT ( 'NONE',  ( 16.75000000000000000, -0.2038245569916320166, 23.22168783648699986 ) ) ;
#12818=CARTESIAN_POINT ( 'NONE',  ( 15.08757311576526128, -0.3152598339554890106, 21.29473909965996015 ) ) ;
#12819=CARTESIAN_POINT ( 'NONE',  ( -14.25000000000000000, -2.500000000000000000, -23.22168783648699986 ) ) ;
#12832=ADVANCED_FACE ( 'NONE', ( #11104 ), #2881, .T. ) ;
#12846=B_SPLINE_CURVE_WITH_KNOTS ( 'NONE', 3,
 ( #1647, #14666, #9931, #9699, #14590, #2728 ),
 .UNSPECIFIED., .F., .F.,
 ( 4, 2, 4 ),
 ( 1.820537833122030991, 2.555393473688635453, 3.290249114255240137 ),
 .UNSPECIFIED. ) ;
#12848=PLANE ( 'NONE',  #8976 ) ;
#12849=ADVANCED_FACE ( 'NONE', ( #13955 ), #5751, .F. ) ;
#12857=DIRECTION ( 'NONE',  ( 0.000000000000000000, 1.000000000000000000, 0.000000000000000000 ) ) ;
#12860=ADVANCED_FACE ( 'NONE', ( #996 ), #10453, .F. ) ;
#12862=DIRECTION ( 'NONE',  ( 0.000000000000000000, 0.000000000000000000, 1.000000000000000000 ) ) ;
#12863=CARTESIAN_POINT ( 'NONE',  ( -15.50000000000000000, -1.037157890325000054, 18.50000000000000000 ) ) ;
#12864=CARTESIAN_POINT ( 'NONE',  ( 15.50000000000000000, -2.500000000000000000, 23.94337567297399971 ) ) ;
#12865=ORIENTED_EDGE ( 'NONE', *, *, #10564, .T. ) ;
#12867=EDGE_CURVE ( 'NONE', #3023, #10723, #2237, .T. ) ;
#12873=ORIENTED_EDGE ( 'NONE', *, *, #13046, .T. ) ;
#12883=CARTESIAN_POINT ( 'NONE',  ( 16.75000000000000000, -0.2038245569916320166, -21.77831216351300014 ) ) ;
#12894=FACE_OUTER_BOUND ( 'NONE', #10508, .T. ) ;
#12903=CARTESIAN_POINT ( 'NONE',  ( -16.75000000000000000, -2.500000000000000000, 21.77831216351300014 ) ) ;
#12904=ORIENTED_EDGE ( 'NONE', *, *, #2580, .T. ) ;
#12909=LINE ( 'NONE', #5562, #10686 ) ;
#12920=CARTESIAN_POINT ( 'NONE',  ( -15.50000000000000000, 998.9628421096749662, -22.50000000000000000 ) ) ;
#12921=AXIS2_PLACEMENT_3D ( 'NONE', #1116, #11663, #11595 ) ;
#12925=CARTESIAN_POINT ( 'NONE',  ( 23.25000000000000000, -5.000000000000000000, 0.000000000000000000 ) ) ;
#12927=VERTEX_POINT ( 'NONE', #14356 ) ;
#12937=AXIS2_PLACEMENT_3D ( 'NONE', #15090, #15164, #6899 ) ;
#12945=VERTEX_POINT ( 'NONE', #2164 ) ;
#12976=CARTESIAN_POINT ( 'NONE',  ( 14.25000000000000000, -0.2038245569916330158, 21.77831216351300014 ) ) ;
#12981=CARTESIAN_POINT ( 'NONE',  ( -23.25000000000000000, -10.00000000000000000, -27.00000000000000000 ) ) ;
#13009=ORIENTED_EDGE ( 'NONE', *, *, #8409, .T. ) ;
#13024=CIRCLE ( 'NONE', #2617, 4.000000000000000000 ) ;
#13030=ORIENTED_EDGE ( 'NONE', *, *, #11728, .F. ) ;
#13035=DIRECTION ( 'NONE',  ( 0.000000000000000000, 0.000000000000000000, 1.000000000000000000 ) ) ;
#13046=EDGE_CURVE ( 'NONE', #3023, #10251, #7020, .T. ) ;
#13064=CARTESIAN_POINT ( 'NONE',  ( 15.50000000000000000, -5.000000000000000000, -22.50000000000000000 ) ) ;
#13066=DIRECTION ( 'NONE',  ( 0.000000000000000000, 1.000000000000000000, 0.000000000000000000 ) ) ;
#13067=CARTESIAN_POINT ( 'NONE',  ( -16.33757311576526305, -0.3152598339554828488, 23.45980260912095616 ) ) ;
#13070=CARTESIAN_POINT ( 'NONE',  ( -15.29686605391142606, -0.2715358723588626733, -21.17390376548178210 ) ) ;
#13084=DIRECTION ( 'NONE',  ( 0.3479852726768751237, 0.000000000000000000, -0.9375000000000004441 ) ) ;
#13087=AXIS2_PLACEMENT_3D ( 'NONE', #8085, #15207, #9394 ) ;
#13090=LINE ( 'NONE', #3451, #7372 ) ;
#13092=SHAPE_DEFINITION_REPRESENTATION ( #626, #2929 ) ;
#13100=DIRECTION ( 'NONE',  ( 0.000000000000000000, 1.000000000000000000, 0.000000000000000000 ) ) ;
#13101=DIRECTION ( 'NONE',  ( 0.000000000000000000, -1.000000000000000000, -0.000000000000000000 ) ) ;
#13107=LINE ( 'NONE', #7365, #10230 ) ;
#13116=DIRECTION ( 'NONE',  ( 0.000000000000000000, 0.000000000000000000, 1.000000000000000000 ) ) ;
#13129=VERTEX_POINT ( 'NONE', #1519 ) ;
#13130=( LENGTH_UNIT ( ) NAMED_UNIT ( * ) SI_UNIT ( .MILLI., .METRE. ) );
#13132=B_SPLINE_CURVE_WITH_KNOTS ( 'NONE', 3,
 ( #2268, #3747, #4761, #9477, #14217, #8407 ),
 .UNSPECIFIED., .F., .F.,
 ( 4, 2, 4 ),
 ( 1.820537833122031213, 2.555393473688635453, 3.290249114255239693 ),
 .UNSPECIFIED. ) ;
#13133=CARTESIAN_POINT ( 'NONE',  ( 14.66434062215688883, -0.3156604612129069731, 21.53909249377453250 ) ) ;
#13136=LINE ( 'NONE', #7236, #1152 ) ;
#13154=FACE_BOUND ( 'NONE', #10052, .T. ) ;
#13159=CYLINDRICAL_SURFACE ( 'NONE', #13315, 4.000000000000000000 ) ;
#13163=VERTEX_POINT ( 'NONE', #13921 ) ;
#13173=LINE ( 'NONE', #7284, #13551 ) ;
#13175=ORIENTED_EDGE ( 'NONE', *, *, #8478, .F. ) ;
#13183=AXIS2_PLACEMENT_3D ( 'NONE', #7185, #98, #7254 ) ;
#13184=DIRECTION ( 'NONE',  ( 0.000000000000000000, 1.000000000000000000, 0.000000000000000000 ) ) ;
#13185=AXIS2_PLACEMENT_3D ( 'NONE', #3727, #6002, #11953 ) ;
#13190=DIRECTION ( 'NONE',  ( -1.284980352575412699E-16, 0.000000000000000000, -1.000000000000000000 ) ) ;
#13193=CARTESIAN_POINT ( 'NONE',  ( -15.50000000000000000, 0.000000000000000000, -22.50000000000000000 ) ) ;
#13195=VERTEX_POINT ( 'NONE', #3293 ) ;
#13198=ORIENTED_EDGE ( 'NONE', *, *, #1070, .T. ) ;
#13207=ADVANCED_FACE ( 'NONE', ( #808 ), #5298, .T. ) ;
#13208=CARTESIAN_POINT ( 'NONE',  ( 15.50000000000000000, -0.2038245569916610489, 21.05662432702600029 ) ) ;
#13216=CARTESIAN_POINT ( 'NONE',  ( -23.24999999999999289, 0.000000000000000000, 27.00000000000000000 ) ) ;
#13228=DIRECTION ( 'NONE',  ( 0.000000000000000000, 1.000000000000000000, 0.000000000000000000 ) ) ;
#13235=AXIS2_PLACEMENT_3D ( 'NONE', #4028, #7686, #535 ) ;
#13269=SURFACE_STYLE_FILL_AREA ( #1309 ) ;
#13275=ORIENTED_EDGE ( 'NONE', *, *, #5474, .F. ) ;
#13278=ORIENTED_EDGE ( 'NONE', *, *, #10279, .F. ) ;
#13279=ORIENTED_EDGE ( 'NONE', *, *, #12297, .F. ) ;
#13281=ORIENTED_EDGE ( 'NONE', *, *, #1359, .F. ) ;
#13295=TOROIDAL_SURFACE ( 'NONE', #7595, 3.299999999999470024, 0.2000000000005275058 ) ;
#13299=EDGE_CURVE ( 'NONE', #14910, #6904, #659, .T. ) ;
#13303=EDGE_CURVE ( 'NONE', #9206, #15023, #11889, .T. ) ;
#13310=DIRECTION ( 'NONE',  ( 0.000000000000000000, 1.000000000000000000, 0.000000000000000000 ) ) ;
#13314=ORIENTED_EDGE ( 'NONE', *, *, #15221, .T. ) ;
#13315=AXIS2_PLACEMENT_3D ( 'NONE', #9645, #1439, #3842 ) ;
#13319=ORIENTED_EDGE ( 'NONE', *, *, #11573, .F. ) ;
#13328=DIRECTION ( 'NONE',  ( -0.9375000000000006661, 0.000000000000000000, -0.3479852726768744020 ) ) ;
#13330=LINE ( 'NONE', #6277, #10353 ) ;
#13343=ORIENTED_EDGE ( 'NONE', *, *, #13714, .T. ) ;
#13344=ORIENTED_EDGE ( 'NONE', *, *, #14370, .F. ) ;
#13354=LINE ( 'NONE', #2711, #9984 ) ;
#13359=VERTEX_POINT ( 'NONE', #15145 ) ;
#13370=CARTESIAN_POINT ( 'NONE',  ( -15.50000000000000000, -0.2038245569916614930, -21.05662432702600029 ) ) ;
#13403=DIRECTION ( 'NONE',  ( -0.8660254037844482555, 0.000000000000000000, 0.4999999999999831801 ) ) ;
#13414=CARTESIAN_POINT ( 'NONE',  ( 15.50000000000000000, -0.4000000000000000222, 19.00000000000000355 ) ) ;
#13416=EDGE_CURVE ( 'NONE', #3042, #11390, #1812, .T. ) ;
#13419=CARTESIAN_POINT ( 'NONE',  ( 15.50000000000000000, -0.2038245569916604938, -21.05662432702600029 ) ) ;
#13420=DIRECTION ( 'NONE',  ( 0.000000000000000000, 1.000000000000000000, 0.000000000000000000 ) ) ;
#13423=CARTESIAN_POINT ( 'NONE',  ( 15.70366306705350112, -0.2717122460102739390, -23.82579074638668004 ) ) ;
#13428=EDGE_LOOP ( 'NONE', ( #2269, #4172, #11225, #3378 ) ) ;
#13432=CARTESIAN_POINT ( 'NONE',  ( 15.50000000000000000, 998.9628421096749662, 22.50000000000000000 ) ) ;
#13442=CARTESIAN_POINT ( 'NONE',  ( -15.50000000000000000, -2.500000000000000000, 21.05662432702600029 ) ) ;
#13457=LINE ( 'NONE', #5161, #9809 ) ;
#13476=CARTESIAN_POINT ( 'NONE',  ( -15.50000000000000000, -5.000000000000000000, 26.00000000000000000 ) ) ;
#13480=DIRECTION ( 'NONE',  ( 0.000000000000000000, 0.000000000000000000, 1.000000000000000000 ) ) ;
#13490=EDGE_CURVE ( 'NONE', #3055, #3702, #8272, .T. ) ;
#13493=FACE_OUTER_BOUND ( 'NONE', #2930, .T. ) ;
#13499=AXIS2_PLACEMENT_3D ( 'NONE', #4918, #2422, #9396 ) ;
#13505=ORIENTED_EDGE ( 'NONE', *, *, #12388, .F. ) ;
#13509=FACE_OUTER_BOUND ( 'NONE', #11185, .T. ) ;
#13525=MECHANICAL_DESIGN_GEOMETRIC_PRESENTATION_REPRESENTATION('',(#14245),#10038);
#13533=ADVANCED_FACE ( 'NONE', ( #8794 ), #6111, .F. ) ;
#13545=DIRECTION ( 'NONE',  ( -0.4999999999999832356, 0.000000000000000000, 0.8660254037844483666 ) ) ;
#13546=VECTOR ( 'NONE', #123, 1000.000000000000000 ) ;
#13551=VECTOR ( 'NONE', #12008, 1000.000000000000000 ) ;
#13557=CIRCLE ( 'NONE', #656, 0.2000000000005261458 ) ;
#13559=LINE ( 'NONE', #7666, #14488 ) ;
#13577=EDGE_CURVE ( 'NONE', #3702, #3055, #6554, .T. ) ;
#13593=LINE ( 'NONE', #12506, #2901 ) ;
#13599=CARTESIAN_POINT ( 'NONE',  ( 16.74999999999999289, -0.3152037684892571301, 22.25410949791978155 ) ) ;
#13602=ORIENTED_EDGE ( 'NONE', *, *, #4798, .T. ) ;
#13609=ADVANCED_FACE ( 'NONE', ( #5628 ), #10489, .F. ) ;
#13616=ORIENTED_EDGE ( 'NONE', *, *, #8833, .T. ) ;
#13622=ORIENTED_EDGE ( 'NONE', *, *, #4800, .T. ) ;
#13632=DIRECTION ( 'NONE',  ( 1.000000000000000000, -0.000000000000000000, 1.224646799147353207E-16 ) ) ;
#13635=ORIENTED_EDGE ( 'NONE', *, *, #6508, .T. ) ;
#13640=ORIENTED_EDGE ( 'NONE', *, *, #6216, .T. ) ;
#13648=ORIENTED_EDGE ( 'NONE', *, *, #10649, .T. ) ;
#13649=FACE_OUTER_BOUND ( 'NONE', #7386, .T. ) ;
#13657=CARTESIAN_POINT ( 'NONE',  ( -15.50000000000000000, -1.037157890325000054, -22.50000000000000000 ) ) ;
#13659=CARTESIAN_POINT ( 'NONE',  ( -16.75000000000000000, -0.3156864504677194816, 22.25638000318209109 ) ) ;
#13678=AXIS2_PLACEMENT_3D ( 'NONE', #8022, #5644, #9031 ) ;
#13696=DIRECTION ( 'NONE',  ( 0.000000000000000000, 1.000000000000000000, 0.000000000000000000 ) ) ;
#13714=EDGE_CURVE ( 'NONE', #14839, #3939, #4750, .T. ) ;
#13720=DIRECTION ( 'NONE',  ( 0.8660254037844485886, 0.000000000000000000, -0.4999999999999827360 ) ) ;
#13722=FACE_OUTER_BOUND ( 'NONE', #15216, .T. ) ;
#13725=VECTOR ( 'NONE', #10803, 1000.000000000000000 ) ;
#13735=DIRECTION ( 'NONE',  ( 0.000000000000000000, 0.000000000000000000, 1.000000000000000000 ) ) ;
#13745=CARTESIAN_POINT ( 'NONE',  ( 16.75000000000000000, -0.2038245569916320166, 21.77831216351300014 ) ) ;
#13766=LINE ( 'NONE', #5477, #14146 ) ;
#13778=DIRECTION ( 'NONE',  ( 0.000000000000000000, 0.000000000000000000, -1.000000000000000000 ) ) ;
#13779=CIRCLE ( 'NONE', #2134, 4.000000000000000000 ) ;
#13791=TOROIDAL_SURFACE ( 'NONE', #5395, 3.299999999999474909, 0.2000000000005234813 ) ;
#13796=DIRECTION ( 'NONE',  ( 0.000000000000000000, 1.000000000000000000, 0.000000000000000000 ) ) ;
#13798=DIRECTION ( 'NONE',  ( 0.000000000000000000, 0.000000000000000000, 1.000000000000000000 ) ) ;
#13803=ORIENTED_EDGE ( 'NONE', *, *, #4136, .F. ) ;
#13814=DIRECTION ( 'NONE',  ( 1.060575238724892987E-16, 0.5000000000000199840, -0.8660254037844271613 ) ) ;
#13817=VECTOR ( 'NONE', #10561, 1000.000000000000000 ) ;
#13821=CARTESIAN_POINT ( 'NONE',  ( 15.70313394608856683, -0.2715358723588608414, -21.17390376548178210 ) ) ;
#13822=CARTESIAN_POINT ( 'NONE',  ( -15.70366306705059323, -0.2717122460101009662, -21.17420925361163953 ) ) ;
#13829=FACE_OUTER_BOUND ( 'NONE', #4689, .T. ) ;
#13836=CARTESIAN_POINT ( 'NONE',  ( 16.75000000000000000, -2.500000000000000000, -21.77831216351300014 ) ) ;
#13849=DIRECTION ( 'NONE',  ( 0.000000000000000000, 1.000000000000000000, 0.000000000000000000 ) ) ;
#13850=CARTESIAN_POINT ( 'NONE',  ( 15.50000000000000000, -5.000000000000000000, 22.50000000000000000 ) ) ;
#13852=CARTESIAN_POINT ( 'NONE',  ( -31.00000000000000000, -2.500000000000000000, 45.00000000000000000 ) ) ;
#13853=ORIENTED_EDGE ( 'NONE', *, *, #2193, .T. ) ;
#13854=SURFACE_STYLE_USAGE ( .BOTH. , #7953 ) ;
#13857=EDGE_CURVE ( 'NONE', #10251, #12753, #11029, .T. ) ;
#13861=B_SPLINE_CURVE_WITH_KNOTS ( 'NONE', 3,
 ( #8391, #5, #76, #7088, #2182, #11645 ),
 .UNSPECIFIED., .F., .F.,
 ( 4, 2, 4 ),
 ( 0.0002380763768129734448, 0.7291065797294589146, 1.457975083082104995 ),
 .UNSPECIFIED. ) ;
#13870=VERTEX_POINT ( 'NONE', #5147 ) ;
#13892=EDGE_CURVE ( 'NONE', #6831, #9509, #579, .T. ) ;
#13894=DIRECTION ( 'NONE',  ( 1.000000000000000000, 0.000000000000000000, 0.000000000000000000 ) ) ;
#13903=DIRECTION ( 'NONE',  ( -0.4999999999999832356, 0.000000000000000000, -0.8660254037844483666 ) ) ;
#13909=ORIENTED_EDGE ( 'NONE', *, *, #6508, .F. ) ;
#13921=CARTESIAN_POINT ( 'NONE',  ( -15.50000000000000000, -0.2038245569916614930, -21.05662432702600029 ) ) ;
#13932=AXIS2_PLACEMENT_3D ( 'NONE', #14940, #4104, #12483 ) ;
#13938=PLANE ( 'NONE',  #8471 ) ;
#13946=ORIENTED_EDGE ( 'NONE', *, *, #345, .T. ) ;
#13950=CARTESIAN_POINT ( 'NONE',  ( 15.50000000000000000, 998.9628421096749662, -22.50000000000000000 ) ) ;
#13953=DIRECTION ( 'NONE',  ( 0.000000000000000000, 0.000000000000000000, 1.000000000000000000 ) ) ;
#13955=FACE_OUTER_BOUND ( 'NONE', #2308, .T. ) ;
#13973=FILL_AREA_STYLE ('',( #14284 ) ) ;
#13975=CARTESIAN_POINT ( 'NONE',  ( 15.50000000000000000, -5.000000000000000000, 26.50000000000000000 ) ) ;
#13980=DIRECTION ( 'NONE',  ( 0.000000000000000000, 1.000000000000000000, 0.000000000000000000 ) ) ;
#13981=EDGE_CURVE ( 'NONE', #3702, #14751, #3961, .T. ) ;
#13996=DIRECTION ( 'NONE',  ( 0.000000000000000000, 1.000000000000000000, 0.000000000000000000 ) ) ;
#14005=CLOSED_SHELL ( 'NONE', ( #11152, #3717, #6113, #7377, #10568, #10617, #3557, #11819, #4469, #8967, #14139, #2472, #5940, #3570, #7087 ) ) ;
#14006=ORIENTED_EDGE ( 'NONE', *, *, #12740, .F. ) ;
#14008=SURFACE_STYLE_FILL_AREA ( #15079 ) ;
#14013=DIRECTION ( 'NONE',  ( 0.000000000000000000, 0.000000000000000000, 1.000000000000000000 ) ) ;
#14018=CARTESIAN_POINT ( 'NONE',  ( 15.50000000000000000, 0.000000000000000000, 18.50000000000000000 ) ) ;
#14030=VERTEX_POINT ( 'NONE', #2952 ) ;
#14046=ORIENTED_EDGE ( 'NONE', *, *, #11722, .T. ) ;
#14051=( NAMED_UNIT ( * ) PLANE_ANGLE_UNIT ( ) SI_UNIT ( $, .RADIAN. ) );
#14053=EDGE_CURVE ( 'NONE', #7246, #1528, #10254, .T. ) ;
#14060=PLANE ( 'NONE',  #4132 ) ;
#14065=EDGE_LOOP ( 'NONE', ( #1438, #4278, #3037, #12788 ) ) ;
#14077=ADVANCED_FACE ( 'NONE', ( #13509 ), #4323, .F. ) ;
#14078=FACE_BOUND ( 'NONE', #2001, .T. ) ;
#14085=FACE_OUTER_BOUND ( 'NONE', #6551, .T. ) ;
#14089=LINE ( 'NONE', #12925, #3603 ) ;
#14094=EDGE_CURVE ( 'NONE', #9286, #4436, #3807, .T. ) ;
#14095=EDGE_CURVE ( 'NONE', #11599, #7739, #7392, .T. ) ;
#14107=ORIENTED_EDGE ( 'NONE', *, *, #9772, .F. ) ;
#14109=PLANE ( 'NONE',  #9756 ) ;
#14120=LINE ( 'NONE', #11569, #9482 ) ;
#14128=CARTESIAN_POINT ( 'NONE',  ( 15.50000000000000000, -2.500000000000000000, 23.94337567297399971 ) ) ;
#14139=ADVANCED_FACE ( 'NONE', ( #7840 ), #10499, .F. ) ;
#14141=ORIENTED_EDGE ( 'NONE', *, *, #339, .T. ) ;
#14146=VECTOR ( 'NONE', #3059, 1000.000000000000114 ) ;
#14154=ORIENTED_EDGE ( 'NONE', *, *, #1553, .F. ) ;
#14156=CIRCLE ( 'NONE', #5749, 3.499999999999999556 ) ;
#14158=ORIENTED_EDGE ( 'NONE', *, *, #9675, .T. ) ;
#14159=AXIS2_PLACEMENT_3D ( 'NONE', #1699, #7829, #7757 ) ;
#14166=VECTOR ( 'NONE', #2515, 1000.000000000000114 ) ;
#14168=DIRECTION ( 'NONE',  ( 0.000000000000000000, 1.000000000000000000, 0.000000000000000000 ) ) ;
#14169=VERTEX_POINT ( 'NONE', #139 ) ;
#14173=AXIS2_PLACEMENT_3D ( 'NONE', #679, #4182, #13720 ) ;
#14176=ORIENTED_EDGE ( 'NONE', *, *, #1553, .T. ) ;
#14186=CARTESIAN_POINT ( 'NONE',  ( -23.25000000000000000, 0.000000000000000000, -27.00000000000000000 ) ) ;
#14187=FACE_OUTER_BOUND ( 'NONE', #11060, .T. ) ;
#14196=EDGE_LOOP ( 'NONE', ( #11167, #4226, #3441, #7903 ) ) ;
#14206=DIRECTION ( 'NONE',  ( 1.000000000000000000, 0.000000000000000000, -1.284980352575412699E-16 ) ) ;
#14214=CARTESIAN_POINT ( 'NONE',  ( -15.50000000000000000, -5.000000000000000000, -19.00000000000000000 ) ) ;
#14217=CARTESIAN_POINT ( 'NONE',  ( -16.75000000000000000, -0.2714405302574915413, -22.01253933645463334 ) ) ;
#14223=CARTESIAN_POINT ( 'NONE',  ( 0.000000000000000000, -5.000000000000000000, 0.000000000000000000 ) ) ;
#14233=ORIENTED_EDGE ( 'NONE', *, *, #3459, .T. ) ;
#14239=ADVANCED_FACE ( 'NONE', ( #9597 ), #6980, .F. ) ;
#14242=LINE ( 'NONE', #1289, #11114 ) ;
#14245=STYLED_ITEM ( 'NONE', ( #2287 ), #298 ) ;
#14250=SHAPE_REPRESENTATION_RELATIONSHIP ( 'NONE' , 'NONE' ,  #2929, #3867 ) ;
#14253=CARTESIAN_POINT ( 'NONE',  ( 15.50000000000000000, -0.4000000000000000222, -19.00000000000000355 ) ) ;
#14262=AXIS2_PLACEMENT_3D ( 'NONE', #2998, #13632, #13778 ) ;
#14272=ORIENTED_EDGE ( 'NONE', *, *, #2519, .F. ) ;
#14284=FILL_AREA_STYLE_COLOUR ( '', #6133 ) ;
#14288=DIRECTION ( 'NONE',  ( 0.8660254037844482555, 0.000000000000000000, -0.4999999999999831801 ) ) ;
#14297=ORIENTED_EDGE ( 'NONE', *, *, #8409, .F. ) ;
#14323=DIRECTION ( 'NONE',  ( -0.000000000000000000, 0.000000000000000000, 1.000000000000000000 ) ) ;
#14326=ADVANCED_FACE ( 'NONE', ( #15259 ), #14109, .T. ) ;
#14331=VERTEX_POINT ( 'NONE', #7603 ) ;
#14337=CARTESIAN_POINT ( 'NONE',  ( 15.50000000000000000, 0.000000000000000000, -26.50000000000000000 ) ) ;
#14342=ORIENTED_EDGE ( 'NONE', *, *, #5287, .F. ) ;
#14352=CARTESIAN_POINT ( 'NONE',  ( 30.00000000000000000, -5.000000000000000000, -27.00000000000000000 ) ) ;
#14356=CARTESIAN_POINT ( 'NONE',  ( -16.75000000000000000, -0.2038245569916330158, -23.22168783648699986 ) ) ;
#14368=ORIENTED_EDGE ( 'NONE', *, *, #11121, .F. ) ;
#14370=EDGE_CURVE ( 'NONE', #11286, #1855, #10929, .T. ) ;
#14396=EDGE_LOOP ( 'NONE', ( #12512, #10545 ) ) ;
#14398=ORIENTED_EDGE ( 'NONE', *, *, #8789, .T. ) ;
#14401=( GEOMETRIC_REPRESENTATION_CONTEXT ( 3 ) GLOBAL_UNCERTAINTY_ASSIGNED_CONTEXT ( ( #3904 ) ) GLOBAL_UNIT_ASSIGNED_CONTEXT ( ( #13130, #14051, #2252 ) ) REPRESENTATION_CONTEXT ( 'NONE', 'WORKASPACE' ) );
#14413=ORIENTED_EDGE ( 'NONE', *, *, #2817, .F. ) ;
#14415=VERTEX_POINT ( 'NONE', #594 ) ;
#14418=EDGE_LOOP ( 'NONE', ( #11387, #11971, #11033, #2729, #14438, #14628 ) ) ;
#14420=ORIENTED_EDGE ( 'NONE', *, *, #5948, .T. ) ;
#14423=COLOUR_RGB ( '', 0.40784314, 0.44705882, 0.49803922) ;
#14431=CARTESIAN_POINT ( 'NONE',  ( 15.50000000000000000, -1.037157890325000054, 26.50000000000000000 ) ) ;
#14437=DIRECTION ( 'NONE',  ( 0.000000000000000000, 0.000000000000000000, 1.000000000000000000 ) ) ;
#14438=ORIENTED_EDGE ( 'NONE', *, *, #10272, .T. ) ;
#14449=CARTESIAN_POINT ( 'NONE',  ( -15.50000000000000000, -0.2038245569916614930, 21.05662432702600029 ) ) ;
#14478=LINE ( 'NONE', #2302, #11753 ) ;
#14479=VECTOR ( 'NONE', #4292, 1000.000000000000114 ) ;
#14488=VECTOR ( 'NONE', #2921, 1000.000000000000114 ) ;
#14490=CARTESIAN_POINT ( 'NONE',  ( 15.29633693294940677, -0.2717122460100966919, -21.17420925361164308 ) ) ;
#14497=ORIENTED_EDGE ( 'NONE', *, *, #13490, .T. ) ;
#14500=DIRECTION ( 'NONE',  ( 0.000000000000000000, 1.000000000000000000, 0.000000000000000000 ) ) ;
#14507=DIRECTION ( 'NONE',  ( 0.4999999999999827360, 0.000000000000000000, 0.8660254037844485886 ) ) ;
#14514=CONICAL_SURFACE ( 'NONE', #9052, 1732.050807568789651, 1.047197551196575871 ) ;
#14531=CARTESIAN_POINT ( 'NONE',  ( 15.50000000000000000, -0.1999999999999999556, 21.05000000000000426 ) ) ;
#14547=FACE_OUTER_BOUND ( 'NONE', #4609, .T. ) ;
#14557=ADVANCED_FACE ( 'NONE', ( #11611, #4177 ), #8901, .T. ) ;
#14558=ORIENTED_EDGE ( 'NONE', *, *, #11337, .F. ) ;
#14566=CARTESIAN_POINT ( 'NONE',  ( -15.50000000000000000, -0.1999999999999999556, -22.50000000000000000 ) ) ;
#14570=CARTESIAN_POINT ( 'NONE',  ( -23.24999999999999289, -10.00000000000000000, 27.00000000000000000 ) ) ;
#14572=LINE ( 'NONE', #5043, #4544 ) ;
#14578=ORIENTED_EDGE ( 'NONE', *, *, #6444, .F. ) ;
#14581=DIRECTION ( 'NONE',  ( 0.000000000000000000, 1.000000000000000000, 0.000000000000000000 ) ) ;
#14588=CARTESIAN_POINT ( 'NONE',  ( 15.50000000000000000, -1.037157890325000054, 19.00000000000000000 ) ) ;
#14590=CARTESIAN_POINT ( 'NONE',  ( 16.75000000000000000, -0.2714405302574892098, -22.98746066354537376 ) ) ;
#14617=LINE ( 'NONE', #11652, #12254 ) ;
#14620=DIRECTION ( 'NONE',  ( 0.000000000000000000, 0.000000000000000000, 1.000000000000000000 ) ) ;
#14626=CARTESIAN_POINT ( 'NONE',  ( 16.75000000000000000, -2.500000000000000000, 23.22168783648699986 ) ) ;
#14628=ORIENTED_EDGE ( 'NONE', *, *, #5748, .T. ) ;
#14644=PLANE ( 'NONE',  #11745 ) ;
#14645=ORIENTED_EDGE ( 'NONE', *, *, #10564, .F. ) ;
#14646=AXIS2_PLACEMENT_3D ( 'NONE', #4458, #10412, #3371 ) ;
#14649=ORIENTED_EDGE ( 'NONE', *, *, #9024, .F. ) ;
#14656=CARTESIAN_POINT ( 'NONE',  ( 15.50000000000000000, -1.037157890325000054, 22.50000000000000000 ) ) ;
#14658=CARTESIAN_POINT ( 'NONE',  ( 14.24999999999999822, -0.3152037684892591285, -22.25410949791979220 ) ) ;
#14664=CARTESIAN_POINT ( 'NONE',  ( -15.50000000000000000, 0.000000000000000000, 18.50000000000000000 ) ) ;
#14666=CARTESIAN_POINT ( 'NONE',  ( 16.75000000000000355, -0.2715193793361411756, -22.01281590054916038 ) ) ;
#14671=ORIENTED_EDGE ( 'NONE', *, *, #1359, .T. ) ;
#14676=DIRECTION ( 'NONE',  ( -0.000000000000000000, 1.000000000000000000, -0.000000000000000000 ) ) ;
#14680=CARTESIAN_POINT ( 'NONE',  ( -16.94999999999999929, -0.2000000000000000111, 22.50000000000000000 ) ) ;
#14681=CARTESIAN_POINT ( 'NONE',  ( -15.50000000000000000, -5.000000000000000000, 22.50000000000000000 ) ) ;
#14687=EDGE_LOOP ( 'NONE', ( #1999, #14578, #7543, #5069 ) ) ;
#14696=AXIS2_PLACEMENT_3D ( 'NONE', #12295, #13545, #3838 ) ;
#14697=CARTESIAN_POINT ( 'NONE',  ( -15.50000000000000000, -1.037157890325000054, 22.50000000000000000 ) ) ;
#14701=PLANE ( 'NONE',  #1280 ) ;
#14704=ORIENTED_EDGE ( 'NONE', *, *, #4800, .F. ) ;
#14715=FACE_OUTER_BOUND ( 'NONE', #11741, .T. ) ;
#14716=CARTESIAN_POINT ( 'NONE',  ( -14.24999999999999822, -0.3152037684892585179, -22.74589050208021135 ) ) ;
#14718=VECTOR ( 'NONE', #2865, 1000.000000000000114 ) ;
#14720=CARTESIAN_POINT ( 'NONE',  ( -14.25000000000000000, -2.500000000000000000, 21.77831216351300014 ) ) ;
#14722=CARTESIAN_POINT ( 'NONE',  ( 16.33757311576526305, -0.3152598339554824047, -23.45980260912095616 ) ) ;
#14731=EDGE_CURVE ( 'NONE', #6904, #541, #13766, .T. ) ;
#14734=FACE_BOUND ( 'NONE', #10569, .T. ) ;
#14737=CARTESIAN_POINT ( 'NONE',  ( -16.75000000000000000, -0.2038245569916330158, 23.22168783648699986 ) ) ;
#14748=ORIENTED_EDGE ( 'NONE', *, *, #13416, .F. ) ;
#14749=VECTOR ( 'NONE', #2525, 1000.000000000000000 ) ;
#14751=VERTEX_POINT ( 'NONE', #1969 ) ;
#14752=CIRCLE ( 'NONE', #10534, 3.299999999999473577 ) ;
#14761=LINE ( 'NONE', #6337, #9309 ) ;
#14779=LINE ( 'NONE', #15075, #1961 ) ;
#14783=FACE_OUTER_BOUND ( 'NONE', #13428, .T. ) ;
#14790=CARTESIAN_POINT ( 'NONE',  ( 23.25000000000000000, -10.00000000000000000, -27.00000000000000000 ) ) ;
#14795=PLANE ( 'NONE',  #14159 ) ;
#14796=AXIS2_PLACEMENT_3D ( 'NONE', #6782, #10329, #7933 ) ;
#14797=ORIENTED_EDGE ( 'NONE', *, *, #4403, .F. ) ;
#14800=ORIENTED_EDGE ( 'NONE', *, *, #11955, .F. ) ;
#14802=ORIENTED_EDGE ( 'NONE', *, *, #14053, .T. ) ;
#14804=EDGE_LOOP ( 'NONE', ( #341, #7268, #13602, #5841 ) ) ;
#14805=DIRECTION ( 'NONE',  ( 0.000000000000000000, 0.000000000000000000, 1.000000000000000000 ) ) ;
#14807=VECTOR ( 'NONE', #13190, 1000.000000000000000 ) ;
#14824=ORIENTED_EDGE ( 'NONE', *, *, #595, .F. ) ;
#14837=ORIENTED_EDGE ( 'NONE', *, *, #12568, .F. ) ;
#14839=VERTEX_POINT ( 'NONE', #7179 ) ;
#14849=DIRECTION ( 'NONE',  ( 0.000000000000000000, 0.000000000000000000, 1.000000000000000000 ) ) ;
#14854=ORIENTED_EDGE ( 'NONE', *, *, #4980, .F. ) ;
#14861=PRESENTATION_STYLE_ASSIGNMENT (( #12332 ) ) ;
#14869=ORIENTED_EDGE ( 'NONE', *, *, #2177, .F. ) ;
#14875=CARTESIAN_POINT ( 'NONE',  ( 14.25000000000000000, -2.500000000000000000, -21.77831216351300014 ) ) ;
#14883=CARTESIAN_POINT ( 'NONE',  ( -16.33757311576526305, -0.3152598339554808504, -21.54019739087904384 ) ) ;
#14890=B_SPLINE_CURVE_WITH_KNOTS ( 'NONE', 3,
 ( #6091, #10802, #13067, #10637, #10882, #12045 ),
 .UNSPECIFIED., .F., .F.,
 ( 4, 2, 4 ),
 ( 0.0002380763768113913770, 0.7291065797294570272, 1.457975083082102774 ),
 .UNSPECIFIED. ) ;
#14893=EDGE_CURVE ( 'NONE', #12927, #11166, #13132, .T. ) ;
#14901=FACE_OUTER_BOUND ( 'NONE', #5442, .T. ) ;
#14903=DIRECTION ( 'NONE',  ( 0.4999999999999827360, 0.000000000000000000, -0.8660254037844485886 ) ) ;
#14906=VERTEX_POINT ( 'NONE', #1425 ) ;
#14907=COLOUR_RGB ( '', 0.08235294, 0.09019608, 0.10196078) ;
#14910=VERTEX_POINT ( 'NONE', #12903 ) ;
#14912=ORIENTED_EDGE ( 'NONE', *, *, #2817, .T. ) ;
#14914=ADVANCED_FACE ( 'NONE', ( #2498 ), #15218, .F. ) ;
#14917=EDGE_CURVE ( 'NONE', #8137, #13129, #14156, .T. ) ;
#14919=( GEOMETRIC_REPRESENTATION_CONTEXT ( 3 ) GLOBAL_UNCERTAINTY_ASSIGNED_CONTEXT ( ( #2970 ) ) GLOBAL_UNIT_ASSIGNED_CONTEXT ( ( #10862, #10782, #146 ) ) REPRESENTATION_CONTEXT ( 'NONE', 'WORKASPACE' ) );
#14924=CARTESIAN_POINT ( 'NONE',  ( -15.50000000000000000, -1.037157890325000054, -22.50000000000000000 ) ) ;
#14940=CARTESIAN_POINT ( 'NONE',  ( -15.50000000000000000, -1.037157890325000054, -22.50000000000000000 ) ) ;
#14941=CARTESIAN_POINT ( 'NONE',  ( 15.50000000000000000, -2.500000000000000000, -23.94337567297399971 ) ) ;
#14942=CARTESIAN_POINT ( 'NONE',  ( 15.50000000000000000, -0.1999999999999999556, -22.50000000000000000 ) ) ;
#14945=VECTOR ( 'NONE', #10284, 1000.000000000000000 ) ;
#14949=EDGE_LOOP ( 'NONE', ( #6849, #10871, #10960, #9567 ) ) ;
#14950=ORIENTED_EDGE ( 'NONE', *, *, #15004, .T. ) ;
#14971=CARTESIAN_POINT ( 'NONE',  ( 16.75000000000000000, -2.500000000000000000, -21.77831216351300014 ) ) ;
#14981=EDGE_LOOP ( 'NONE', ( #1146, #15193, #15251, #8053, #10214, #4647 ) ) ;
#14999=CARTESIAN_POINT ( 'NONE',  ( 15.50000000000000000, -2.500000000000000000, 23.94337567297399971 ) ) ;
#15001=VECTOR ( 'NONE', #14288, 1000.000000000000114 ) ;
#15004=EDGE_CURVE ( 'NONE', #11427, #7228, #4141, .T. ) ;
#15023=VERTEX_POINT ( 'NONE', #5391 ) ;
#15025=VECTOR ( 'NONE', #496, 1000.000000000000000 ) ;
#15028=EDGE_LOOP ( 'NONE', ( #7242, #7374 ) ) ;
#15029=ORIENTED_EDGE ( 'NONE', *, *, #13490, .F. ) ;
#15040=CYLINDRICAL_SURFACE ( 'NONE', #6825, 3.499999999999999556 ) ;
#15041=CARTESIAN_POINT ( 'NONE',  ( 16.54633693294649888, -0.2717122460102533998, -21.66072723692568402 ) ) ;
#15045=ORIENTED_EDGE ( 'NONE', *, *, #805, .F. ) ;
#15048=UNCERTAINTY_MEASURE_WITH_UNIT (LENGTH_MEASURE( 1.000000000000000082E-05 ), #3222, 'distance_accuracy_value', 'NONE');
#15050=CARTESIAN_POINT ( 'NONE',  ( 16.54633693294649532, -0.2717122460102548986, 23.33927276307431598 ) ) ;
#15058=LINE ( 'NONE', #3353, #6575 ) ;
#15062=ORIENTED_EDGE ( 'NONE', *, *, #15306, .F. ) ;
#15075=CARTESIAN_POINT ( 'NONE',  ( -16.75000000000000000, -2.500000000000000000, -23.22168783648699986 ) ) ;
#15076=DIRECTION ( 'NONE',  ( 0.000000000000000000, 0.000000000000000000, 1.000000000000000000 ) ) ;
#15077=DIRECTION ( 'NONE',  ( 0.000000000000000000, 1.000000000000000000, 0.000000000000000000 ) ) ;
#15079=FILL_AREA_STYLE ('',( #9186 ) ) ;
#15090=CARTESIAN_POINT ( 'NONE',  ( -14.25000000000000000, -2.500000000000000000, -23.22168783648699986 ) ) ;
#15091=ORIENTED_EDGE ( 'NONE', *, *, #5287, .T. ) ;
#15115=ORIENTED_EDGE ( 'NONE', *, *, #4658, .F. ) ;
#15139=ORIENTED_EDGE ( 'NONE', *, *, #3660, .F. ) ;
#15143=AXIS2_PLACEMENT_3D ( 'NONE', #9429, #14168, #3545 ) ;
#15145=CARTESIAN_POINT ( 'NONE',  ( 15.50000000000000000, -0.1999999999999999556, 23.94999999999999574 ) ) ;
#15157=AXIS2_PLACEMENT_3D ( 'NONE', #9603, #2550, #3794 ) ;
#15163=DIRECTION ( 'NONE',  ( -1.000000000000000000, 0.000000000000000000, 0.000000000000000000 ) ) ;
#15164=DIRECTION ( 'NONE',  ( 0.4999999999999827360, 0.000000000000000000, -0.8660254037844485886 ) ) ;
#15167=DIRECTION ( 'NONE',  ( -1.000000000000000000, 0.000000000000000000, 0.000000000000000000 ) ) ;
#15168=PRODUCT_DEFINITION ( 'UNKNOWN', '', #11884, #12285 ) ;
#15169=EDGE_CURVE ( 'NONE', #10998, #7322, #938, .T. ) ;
#15174=EDGE_LOOP ( 'NONE', ( #6681, #7014 ) ) ;
#15191=PLANE ( 'NONE',  #6730 ) ;
#15193=ORIENTED_EDGE ( 'NONE', *, *, #11728, .T. ) ;
#15206=ADVANCED_FACE ( 'NONE', ( #13829 ), #4283, .F. ) ;
#15207=DIRECTION ( 'NONE',  ( 0.000000000000000000, 1.000000000000000000, 0.000000000000000000 ) ) ;
#15216=EDGE_LOOP ( 'NONE', ( #12904, #11969, #5670, #2160 ) ) ;
#15218=PLANE ( 'NONE',  #8214 ) ;
#15221=EDGE_CURVE ( 'NONE', #5866, #4720, #1075, .T. ) ;
#15226=AXIS2_PLACEMENT_3D ( 'NONE', #14656, #4041, #6087 ) ;
#15228=VECTOR ( 'NONE', #10228, 1000.000000000000114 ) ;
#15235=CARTESIAN_POINT ( 'NONE',  ( -15.50000000000000000, -0.2038245569916614930, 21.05662432702600029 ) ) ;
#15240=CARTESIAN_POINT ( 'NONE',  ( 0.000000000000000000, -2.500000000000000000, 0.000000000000000000 ) ) ;
#15246=CIRCLE ( 'NONE', #11542, 3.300000002979700753 ) ;
#15247=DIRECTION ( 'NONE',  ( 0.000000000000000000, 1.000000000000000000, 0.000000000000000000 ) ) ;
#15251=ORIENTED_EDGE ( 'NONE', *, *, #3265, .T. ) ;
#15259=FACE_OUTER_BOUND ( 'NONE', #11699, .T. ) ;
#15293=EDGE_LOOP ( 'NONE', ( #14297, #3883, #8328, #9832 ) ) ;
#15302=FACE_OUTER_BOUND ( 'NONE', #5389, .T. ) ;
#15304=DIRECTION ( 'NONE',  ( 0.000000000000000000, 0.000000000000000000, 1.000000000000000000 ) ) ;
#15306=EDGE_CURVE ( 'NONE', #382, #4318, #5266, .T. ) ;
#15311=DIRECTION ( 'NONE',  ( 0.000000000000000000, 1.000000000000000000, 0.000000000000000000 ) ) ;
#15324=FACE_OUTER_BOUND ( 'NONE', #4186, .T. ) ;
#15327=ORIENTED_EDGE ( 'NONE', *, *, #11591, .T. ) ;
ENDSEC;
END-ISO-10303-21;
